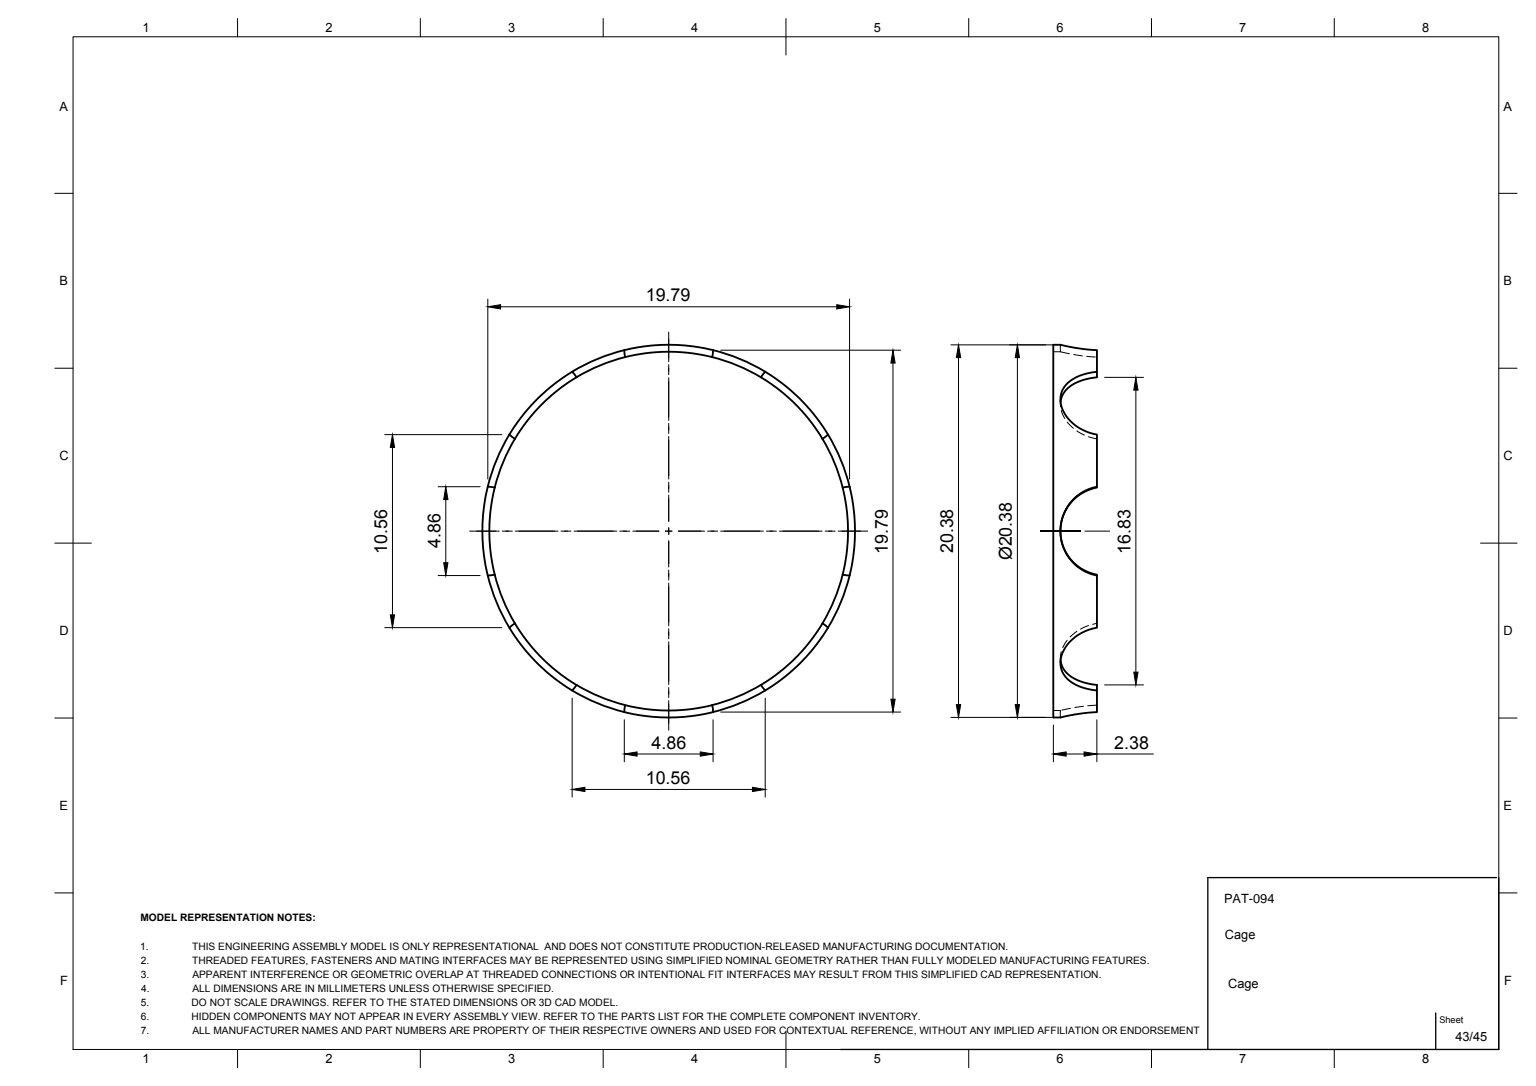
ISO-10303-21;
HEADER;
/* Generated by software containing ST-Developer
 * from STEP Tools, Inc. (www.steptools.com) 
 */

FILE_DESCRIPTION(
/* description */ ('Shaft runout checking stand'),
/* implementation_level */ '2;1');

FILE_NAME(
/* name */ 'Cage.step',
/* time_stamp */ '2026-11-02T21:12:33-08:00',
/* author */ (''),
/* organization */ (''),
/* preprocessor_version */ 'ST-DEVELOPER v20.2',
/* originating_system */ 'Autodesk Translation Framework v15.17.0.0',
/* authorisation */ '');

FILE_SCHEMA (('AUTOMOTIVE_DESIGN { 1 0 10303 214 3 1 1 }'));
ENDSEC;

DATA;
#10=MECHANICAL_DESIGN_GEOMETRIC_PRESENTATION_REPRESENTATION('',(#508),#11748);
#19=SPHERICAL_SURFACE('',#7380,0.247676);
#20=SPHERICAL_SURFACE('',#7396,0.247676);
#21=SPHERICAL_SURFACE('',#7401,0.247676);
#22=SPHERICAL_SURFACE('',#7406,0.247676);
#23=SPHERICAL_SURFACE('',#7411,0.247676);
#24=SPHERICAL_SURFACE('',#7416,0.247676);
#25=SPHERICAL_SURFACE('',#7421,0.247676);
#26=SPHERICAL_SURFACE('',#7429,0.247676);
#335=B_SPLINE_CURVE_WITH_KNOTS('',3,(#11118,#11119,#11120,#11121,#11122,
#11123,#11124,#11125,#11126,#11127,#11128,#11129,#11130,#11131,#11132,#11133,
#11134,#11135,#11136,#11137,#11138,#11139),.UNSPECIFIED.,.F.,.F.,(4,2,2,
2,2,2,2,2,2,2,4),(0.0473477652366656,0.126350602536658,0.189525903804987,
0.252701205073317,0.313298422430275,0.373895639787233,0.434492857144191,
0.495090074501149,0.558265375769478,0.621440677037807,0.7004435143378),
 .UNSPECIFIED.);
#336=B_SPLINE_CURVE_WITH_KNOTS('',3,(#11143,#11144,#11145,#11146,#11147,
#11148,#11149,#11150,#11151,#11152,#11153,#11154,#11155,#11156,#11157,#11158,
#11159,#11160,#11161,#11162,#11163,#11164),.UNSPECIFIED.,.F.,.F.,(4,2,2,
2,2,2,2,2,2,2,4),(0.0464897534940957,0.0852567806515119,0.170513561303024,
0.246687263103517,0.308657850341199,0.370628437578881,0.432599024816563,
0.494569612054245,0.570743313854739,0.656000094506251,0.694767121663666),
 .UNSPECIFIED.);
#337=B_SPLINE_CURVE_WITH_KNOTS('',3,(#11170,#11171,#11172,#11173,#11174,
#11175,#11176,#11177,#11178,#11179,#11180,#11181,#11182,#11183,#11184,#11185,
#11186,#11187,#11188,#11189,#11190,#11191),.UNSPECIFIED.,.F.,.F.,(4,2,2,
2,2,2,2,2,2,2,4),(0.0464897534940957,0.0852567806515118,0.170513561303024,
0.246687263103517,0.308657850341199,0.370628437578881,0.432599024816563,
0.494569612054245,0.570743313854738,0.65600009450625,0.694767121663666),
 .UNSPECIFIED.);
#338=B_SPLINE_CURVE_WITH_KNOTS('',3,(#11195,#11196,#11197,#11198,#11199,
#11200,#11201,#11202,#11203,#11204,#11205,#11206,#11207,#11208,#11209,#11210,
#11211,#11212,#11213,#11214,#11215,#11216),.UNSPECIFIED.,.F.,.F.,(4,2,2,
2,2,2,2,2,2,2,4),(0.0464897534940957,0.0852567806515119,0.170513561303024,
0.246687263103517,0.308657850341199,0.370628437578881,0.432599024816563,
0.494569612054245,0.570743313854739,0.656000094506251,0.694767121663666),
 .UNSPECIFIED.);
#339=B_SPLINE_CURVE_WITH_KNOTS('',3,(#11220,#11221,#11222,#11223,#11224,
#11225,#11226,#11227,#11228,#11229,#11230,#11231),.UNSPECIFIED.,.F.,.F.,
(4,2,2,2,2,4),(0.0464897534940957,0.0852567806515119,0.170513561303024,
0.246687263103517,0.308657850341199,0.370628437578881),.UNSPECIFIED.);
#340=B_SPLINE_CURVE_WITH_KNOTS('',3,(#11236,#11237,#11238,#11239,#11240,
#11241,#11242,#11243,#11244,#11245,#11246,#11247),.UNSPECIFIED.,.F.,.F.,
(4,2,2,2,2,4),(0.370628437578881,0.432599024816563,0.494569612054245,0.570743313854738,
0.65600009450625,0.694767121663666),.UNSPECIFIED.);
#341=B_SPLINE_CURVE_WITH_KNOTS('',3,(#11251,#11252,#11253,#11254,#11255,
#11256,#11257,#11258,#11259,#11260,#11261,#11262,#11263,#11264,#11265,#11266,
#11267,#11268,#11269,#11270,#11271,#11272),.UNSPECIFIED.,.F.,.F.,(4,2,2,
2,2,2,2,2,2,2,4),(0.0464897534940957,0.0852567806515121,0.170513561303024,
0.246687263103518,0.308657850341199,0.370628437578881,0.432599024816563,
0.494569612054245,0.570743313854738,0.65600009450625,0.694767121663666),
 .UNSPECIFIED.);
#342=B_SPLINE_CURVE_WITH_KNOTS('',3,(#11276,#11277,#11278,#11279,#11280,
#11281,#11282,#11283,#11284,#11285,#11286,#11287,#11288,#11289,#11290,#11291,
#11292,#11293,#11294,#11295,#11296,#11297),.UNSPECIFIED.,.F.,.F.,(4,2,2,
2,2,2,2,2,2,2,4),(0.0464897534940957,0.0852567806515119,0.170513561303024,
0.246687263103517,0.308657850341199,0.370628437578881,0.432599024816563,
0.494569612054245,0.570743313854738,0.65600009450625,0.694767121663667),
 .UNSPECIFIED.);
#343=B_SPLINE_CURVE_WITH_KNOTS('',3,(#11301,#11302,#11303,#11304,#11305,
#11306,#11307,#11308,#11309,#11310,#11311,#11312,#11313,#11314,#11315,#11316,
#11317,#11318,#11319,#11320,#11321,#11322),.UNSPECIFIED.,.F.,.F.,(4,2,2,
2,2,2,2,2,2,2,4),(0.0464897534940957,0.0852567806515119,0.170513561303024,
0.246687263103517,0.308657850341199,0.370628437578881,0.432599024816563,
0.494569612054245,0.570743313854738,0.65600009450625,0.694767121663666),
 .UNSPECIFIED.);
#344=B_SPLINE_CURVE_WITH_KNOTS('',3,(#11326,#11327,#11328,#11329,#11330,
#11331,#11332,#11333,#11334,#11335,#11336,#11337,#11338,#11339,#11340,#11341,
#11342,#11343,#11344,#11345,#11346,#11347),.UNSPECIFIED.,.F.,.F.,(4,2,2,
2,2,2,2,2,2,2,4),(0.0464897534940957,0.0852567806515119,0.170513561303024,
0.246687263103517,0.308657850341199,0.370628437578881,0.432599024816563,
0.494569612054245,0.570743313854739,0.656000094506251,0.694767121663667),
 .UNSPECIFIED.);
#345=B_SPLINE_CURVE_WITH_KNOTS('',3,(#11355,#11356,#11357,#11358,#11359,
#11360,#11361,#11362,#11363,#11364,#11365,#11366,#11367,#11368,#11369,#11370,
#11371,#11372,#11373,#11374,#11375,#11376),.UNSPECIFIED.,.F.,.F.,(4,2,2,
2,2,2,2,2,2,2,4),(0.0473477652366656,0.126350602536658,0.189525903804987,
0.252701205073316,0.313298422430274,0.373895639787232,0.434492857144191,
0.495090074501149,0.558265375769478,0.621440677037807,0.7004435143378),
 .UNSPECIFIED.);
#346=B_SPLINE_CURVE_WITH_KNOTS('',3,(#11384,#11385,#11386,#11387,#11388,
#11389,#11390,#11391,#11392,#11393,#11394,#11395,#11396,#11397,#11398,#11399,
#11400,#11401,#11402,#11403,#11404,#11405),.UNSPECIFIED.,.F.,.F.,(4,2,2,
2,2,2,2,2,2,2,4),(0.0473477652366656,0.126350602536658,0.189525903804987,
0.252701205073317,0.313298422430275,0.373895639787233,0.434492857144191,
0.495090074501149,0.558265375769478,0.621440677037807,0.7004435143378),
 .UNSPECIFIED.);
#347=B_SPLINE_CURVE_WITH_KNOTS('',3,(#11414,#11415,#11416,#11417,#11418,
#11419,#11420,#11421,#11422,#11423,#11424,#11425),.UNSPECIFIED.,.F.,.F.,
(4,2,2,2,2,4),(0.0473477652366656,0.126350602536658,0.189525903804987,0.252701205073316,
0.313298422430275,0.373895639787233),.UNSPECIFIED.);
#348=B_SPLINE_CURVE_WITH_KNOTS('',3,(#11427,#11428,#11429,#11430,#11431,
#11432,#11433,#11434,#11435,#11436,#11437,#11438),.UNSPECIFIED.,.F.,.F.,
(4,2,2,2,2,4),(0.373895639787233,0.434492857144191,0.495090074501149,0.558265375769478,
0.621440677037807,0.7004435143378),.UNSPECIFIED.);
#349=B_SPLINE_CURVE_WITH_KNOTS('',3,(#11445,#11446,#11447,#11448,#11449,
#11450,#11451,#11452,#11453,#11454,#11455,#11456,#11457,#11458,#11459,#11460,
#11461,#11462,#11463,#11464,#11465,#11466),.UNSPECIFIED.,.F.,.F.,(4,2,2,
2,2,2,2,2,2,2,4),(0.0473477652366656,0.126350602536658,0.189525903804987,
0.252701205073316,0.313298422430275,0.373895639787233,0.434492857144191,
0.495090074501149,0.558265375769478,0.621440677037807,0.7004435143378),
 .UNSPECIFIED.);
#350=B_SPLINE_CURVE_WITH_KNOTS('',3,(#11474,#11475,#11476,#11477,#11478,
#11479,#11480,#11481,#11482,#11483,#11484,#11485,#11486,#11487,#11488,#11489,
#11490,#11491,#11492,#11493,#11494,#11495),.UNSPECIFIED.,.F.,.F.,(4,2,2,
2,2,2,2,2,2,2,4),(0.0473477652366656,0.126350602536658,0.189525903804987,
0.252701205073317,0.313298422430275,0.373895639787233,0.434492857144191,
0.495090074501149,0.558265375769478,0.621440677037807,0.7004435143378),
 .UNSPECIFIED.);
#351=B_SPLINE_CURVE_WITH_KNOTS('',3,(#11503,#11504,#11505,#11506,#11507,
#11508,#11509,#11510,#11511,#11512,#11513,#11514,#11515,#11516,#11517,#11518,
#11519,#11520,#11521,#11522,#11523,#11524),.UNSPECIFIED.,.F.,.F.,(4,2,2,
2,2,2,2,2,2,2,4),(0.0473477652366656,0.126350602536658,0.189525903804987,
0.252701205073316,0.313298422430275,0.373895639787233,0.434492857144191,
0.495090074501149,0.558265375769478,0.621440677037807,0.7004435143378),
 .UNSPECIFIED.);
#352=B_SPLINE_CURVE_WITH_KNOTS('',3,(#11533,#11534,#11535,#11536,#11537,
#11538,#11539,#11540,#11541,#11542,#11543,#11544,#11545,#11546,#11547,#11548,
#11549,#11550,#11551,#11552,#11553,#11554),.UNSPECIFIED.,.F.,.F.,(4,2,2,
2,2,2,2,2,2,2,4),(0.0473477652366656,0.126350602536658,0.189525903804987,
0.252701205073317,0.313298422430275,0.373895639787233,0.434492857144191,
0.495090074501149,0.558265375769478,0.621440677037807,0.7004435143378),
 .UNSPECIFIED.);
#415=SHAPE_REPRESENTATION_RELATIONSHIP('SRR','None',#11967,#458);
#458=ADVANCED_BREP_SHAPE_REPRESENTATION('',(#556),#11743);
#508=STYLED_ITEM('',(#12169),#556);
#556=MANIFOLD_SOLID_BREP('Continuous crown cage',#6254);
#662=FACE_BOUND('',#1853,.T.);
#884=CIRCLE('',#7381,0.243053047864041);
#885=CIRCLE('',#7382,0.243053047864041);
#886=CIRCLE('',#7384,1.019052);
#887=CIRCLE('',#7385,1.019052);
#888=CIRCLE('',#7386,1.019052);
#889=CIRCLE('',#7387,1.019052);
#890=CIRCLE('',#7388,1.019052);
#891=CIRCLE('',#7389,1.019052);
#892=CIRCLE('',#7390,1.019052);
#893=CIRCLE('',#7391,1.019052);
#894=CIRCLE('',#7392,1.019052);
#895=CIRCLE('',#7394,0.980948);
#896=CIRCLE('',#7395,0.243053047864041);
#897=CIRCLE('',#7397,0.243053047864041);
#898=CIRCLE('',#7399,0.980948);
#899=CIRCLE('',#7400,0.243053047864041);
#900=CIRCLE('',#7402,0.243053047864041);
#901=CIRCLE('',#7404,0.980948);
#902=CIRCLE('',#7405,0.243053047864041);
#903=CIRCLE('',#7407,0.243053047864041);
#904=CIRCLE('',#7409,0.980948);
#905=CIRCLE('',#7410,0.243053047864041);
#906=CIRCLE('',#7412,0.243053047864041);
#907=CIRCLE('',#7414,0.980948);
#908=CIRCLE('',#7415,0.243053047864041);
#909=CIRCLE('',#7417,0.243053047864041);
#910=CIRCLE('',#7419,0.980948);
#911=CIRCLE('',#7420,0.243053047864041);
#912=CIRCLE('',#7422,0.243053047864041);
#913=CIRCLE('',#7424,0.980948);
#914=CIRCLE('',#7425,0.980948);
#915=CIRCLE('',#7426,0.980948);
#916=CIRCLE('',#7428,0.243053047864041);
#917=CIRCLE('',#7430,0.243053047864041);
#1026=CYLINDRICAL_SURFACE('',#7383,1.019052);
#1027=CYLINDRICAL_SURFACE('',#7423,0.980948);
#1367=FACE_OUTER_BOUND('',#1835,.T.);
#1368=FACE_OUTER_BOUND('',#1836,.T.);
#1369=FACE_OUTER_BOUND('',#1837,.T.);
#1370=FACE_OUTER_BOUND('',#1838,.T.);
#1371=FACE_OUTER_BOUND('',#1839,.T.);
#1372=FACE_OUTER_BOUND('',#1840,.T.);
#1373=FACE_OUTER_BOUND('',#1841,.T.);
#1374=FACE_OUTER_BOUND('',#1842,.T.);
#1375=FACE_OUTER_BOUND('',#1843,.T.);
#1376=FACE_OUTER_BOUND('',#1844,.T.);
#1377=FACE_OUTER_BOUND('',#1845,.T.);
#1378=FACE_OUTER_BOUND('',#1846,.T.);
#1379=FACE_OUTER_BOUND('',#1847,.T.);
#1380=FACE_OUTER_BOUND('',#1848,.T.);
#1381=FACE_OUTER_BOUND('',#1849,.T.);
#1382=FACE_OUTER_BOUND('',#1850,.T.);
#1383=FACE_OUTER_BOUND('',#1851,.T.);
#1384=FACE_OUTER_BOUND('',#1852,.T.);
#1385=FACE_OUTER_BOUND('',#1854,.T.);
#1835=EDGE_LOOP('',(#5436,#5437,#5438,#5439));
#1836=EDGE_LOOP('',(#5440,#5441,#5442,#5443,#5444,#5445,#5446,#5447,#5448,
#5449,#5450,#5451,#5452,#5453,#5454,#5455,#5456,#5457,#5458,#5459));
#1837=EDGE_LOOP('',(#5460,#5461,#5462,#5463));
#1838=EDGE_LOOP('',(#5464,#5465,#5466,#5467));
#1839=EDGE_LOOP('',(#5468,#5469,#5470,#5471));
#1840=EDGE_LOOP('',(#5472,#5473,#5474,#5475));
#1841=EDGE_LOOP('',(#5476,#5477,#5478,#5479));
#1842=EDGE_LOOP('',(#5480,#5481,#5482,#5483,#5484,#5485));
#1843=EDGE_LOOP('',(#5486,#5487,#5488,#5489));
#1844=EDGE_LOOP('',(#5490,#5491,#5492,#5493));
#1845=EDGE_LOOP('',(#5494,#5495,#5496,#5497));
#1846=EDGE_LOOP('',(#5498,#5499,#5500,#5501));
#1847=EDGE_LOOP('',(#5502,#5503,#5504,#5505));
#1848=EDGE_LOOP('',(#5506,#5507,#5508,#5509));
#1849=EDGE_LOOP('',(#5510,#5511,#5512,#5513,#5514,#5515,#5516,#5517,#5518,
#5519,#5520,#5521,#5522,#5523,#5524,#5525,#5526,#5527,#5528,#5529));
#1850=EDGE_LOOP('',(#5530,#5531,#5532,#5533));
#1851=EDGE_LOOP('',(#5534,#5535,#5536,#5537));
#1852=EDGE_LOOP('',(#5538));
#1853=EDGE_LOOP('',(#5539));
#1854=EDGE_LOOP('',(#5540,#5541,#5542,#5543));
#2340=LINE('',#11233,#2807);
#2341=LINE('',#11529,#2808);
#2807=VECTOR('',#9253,1.019052);
#2808=VECTOR('',#9330,0.980948);
#3274=VERTEX_POINT('',#11116);
#3275=VERTEX_POINT('',#11117);
#3276=VERTEX_POINT('',#11140);
#3277=VERTEX_POINT('',#11142);
#3278=VERTEX_POINT('',#11167);
#3279=VERTEX_POINT('',#11169);
#3280=VERTEX_POINT('',#11192);
#3281=VERTEX_POINT('',#11194);
#3282=VERTEX_POINT('',#11217);
#3283=VERTEX_POINT('',#11219);
#3284=VERTEX_POINT('',#11232);
#3285=VERTEX_POINT('',#11235);
#3286=VERTEX_POINT('',#11248);
#3287=VERTEX_POINT('',#11250);
#3288=VERTEX_POINT('',#11273);
#3289=VERTEX_POINT('',#11275);
#3290=VERTEX_POINT('',#11298);
#3291=VERTEX_POINT('',#11300);
#3292=VERTEX_POINT('',#11323);
#3293=VERTEX_POINT('',#11325);
#3294=VERTEX_POINT('',#11350);
#3295=VERTEX_POINT('',#11354);
#3296=VERTEX_POINT('',#11379);
#3297=VERTEX_POINT('',#11383);
#3298=VERTEX_POINT('',#11408);
#3299=VERTEX_POINT('',#11412);
#3300=VERTEX_POINT('',#11413);
#3301=VERTEX_POINT('',#11440);
#3302=VERTEX_POINT('',#11444);
#3303=VERTEX_POINT('',#11469);
#3304=VERTEX_POINT('',#11473);
#3305=VERTEX_POINT('',#11498);
#3306=VERTEX_POINT('',#11502);
#3307=VERTEX_POINT('',#11527);
#3308=VERTEX_POINT('',#11530);
#3309=VERTEX_POINT('',#11532);
#4004=EDGE_CURVE('',#3274,#3275,#335,.T.);
#4005=EDGE_CURVE('',#3276,#3274,#884,.T.);
#4006=EDGE_CURVE('',#3277,#3276,#336,.T.);
#4007=EDGE_CURVE('',#3275,#3277,#885,.T.);
#4008=EDGE_CURVE('',#3278,#3276,#886,.T.);
#4009=EDGE_CURVE('',#3278,#3279,#337,.T.);
#4010=EDGE_CURVE('',#3280,#3279,#887,.T.);
#4011=EDGE_CURVE('',#3280,#3281,#338,.T.);
#4012=EDGE_CURVE('',#3282,#3281,#888,.T.);
#4013=EDGE_CURVE('',#3282,#3283,#339,.T.);
#4014=EDGE_CURVE('',#3283,#3284,#2340,.T.);
#4015=EDGE_CURVE('',#3284,#3284,#889,.T.);
#4016=EDGE_CURVE('',#3283,#3285,#340,.T.);
#4017=EDGE_CURVE('',#3286,#3285,#890,.T.);
#4018=EDGE_CURVE('',#3286,#3287,#341,.T.);
#4019=EDGE_CURVE('',#3288,#3287,#891,.T.);
#4020=EDGE_CURVE('',#3288,#3289,#342,.T.);
#4021=EDGE_CURVE('',#3290,#3289,#892,.T.);
#4022=EDGE_CURVE('',#3290,#3291,#343,.T.);
#4023=EDGE_CURVE('',#3292,#3291,#893,.T.);
#4024=EDGE_CURVE('',#3292,#3293,#344,.T.);
#4025=EDGE_CURVE('',#3277,#3293,#894,.T.);
#4026=EDGE_CURVE('',#3274,#3294,#895,.T.);
#4027=EDGE_CURVE('',#3294,#3278,#896,.T.);
#4028=EDGE_CURVE('',#3295,#3294,#345,.T.);
#4029=EDGE_CURVE('',#3279,#3295,#897,.T.);
#4030=EDGE_CURVE('',#3295,#3296,#898,.T.);
#4031=EDGE_CURVE('',#3296,#3280,#899,.T.);
#4032=EDGE_CURVE('',#3297,#3296,#346,.T.);
#4033=EDGE_CURVE('',#3281,#3297,#900,.T.);
#4034=EDGE_CURVE('',#3297,#3298,#901,.T.);
#4035=EDGE_CURVE('',#3298,#3282,#902,.T.);
#4036=EDGE_CURVE('',#3299,#3300,#347,.T.);
#4037=EDGE_CURVE('',#3285,#3299,#903,.T.);
#4038=EDGE_CURVE('',#3300,#3298,#348,.T.);
#4039=EDGE_CURVE('',#3299,#3301,#904,.T.);
#4040=EDGE_CURVE('',#3301,#3286,#905,.T.);
#4041=EDGE_CURVE('',#3302,#3301,#349,.T.);
#4042=EDGE_CURVE('',#3287,#3302,#906,.T.);
#4043=EDGE_CURVE('',#3302,#3303,#907,.T.);
#4044=EDGE_CURVE('',#3303,#3288,#908,.T.);
#4045=EDGE_CURVE('',#3304,#3303,#350,.T.);
#4046=EDGE_CURVE('',#3289,#3304,#909,.T.);
#4047=EDGE_CURVE('',#3304,#3305,#910,.T.);
#4048=EDGE_CURVE('',#3305,#3290,#911,.T.);
#4049=EDGE_CURVE('',#3306,#3305,#351,.T.);
#4050=EDGE_CURVE('',#3291,#3306,#912,.T.);
#4051=EDGE_CURVE('',#3307,#3307,#913,.T.);
#4052=EDGE_CURVE('',#3307,#3300,#2341,.T.);
#4053=EDGE_CURVE('',#3308,#3275,#914,.T.);
#4054=EDGE_CURVE('',#3308,#3309,#352,.T.);
#4055=EDGE_CURVE('',#3306,#3309,#915,.T.);
#4056=EDGE_CURVE('',#3293,#3308,#916,.T.);
#4057=EDGE_CURVE('',#3309,#3292,#917,.T.);
#5436=ORIENTED_EDGE('',*,*,#4004,.F.);
#5437=ORIENTED_EDGE('',*,*,#4005,.F.);
#5438=ORIENTED_EDGE('',*,*,#4006,.F.);
#5439=ORIENTED_EDGE('',*,*,#4007,.F.);
#5440=ORIENTED_EDGE('',*,*,#4006,.T.);
#5441=ORIENTED_EDGE('',*,*,#4008,.F.);
#5442=ORIENTED_EDGE('',*,*,#4009,.T.);
#5443=ORIENTED_EDGE('',*,*,#4010,.F.);
#5444=ORIENTED_EDGE('',*,*,#4011,.T.);
#5445=ORIENTED_EDGE('',*,*,#4012,.F.);
#5446=ORIENTED_EDGE('',*,*,#4013,.T.);
#5447=ORIENTED_EDGE('',*,*,#4014,.T.);
#5448=ORIENTED_EDGE('',*,*,#4015,.F.);
#5449=ORIENTED_EDGE('',*,*,#4014,.F.);
#5450=ORIENTED_EDGE('',*,*,#4016,.T.);
#5451=ORIENTED_EDGE('',*,*,#4017,.F.);
#5452=ORIENTED_EDGE('',*,*,#4018,.T.);
#5453=ORIENTED_EDGE('',*,*,#4019,.F.);
#5454=ORIENTED_EDGE('',*,*,#4020,.T.);
#5455=ORIENTED_EDGE('',*,*,#4021,.F.);
#5456=ORIENTED_EDGE('',*,*,#4022,.T.);
#5457=ORIENTED_EDGE('',*,*,#4023,.F.);
#5458=ORIENTED_EDGE('',*,*,#4024,.T.);
#5459=ORIENTED_EDGE('',*,*,#4025,.F.);
#5460=ORIENTED_EDGE('',*,*,#4005,.T.);
#5461=ORIENTED_EDGE('',*,*,#4026,.T.);
#5462=ORIENTED_EDGE('',*,*,#4027,.T.);
#5463=ORIENTED_EDGE('',*,*,#4008,.T.);
#5464=ORIENTED_EDGE('',*,*,#4028,.F.);
#5465=ORIENTED_EDGE('',*,*,#4029,.F.);
#5466=ORIENTED_EDGE('',*,*,#4009,.F.);
#5467=ORIENTED_EDGE('',*,*,#4027,.F.);
#5468=ORIENTED_EDGE('',*,*,#4029,.T.);
#5469=ORIENTED_EDGE('',*,*,#4030,.T.);
#5470=ORIENTED_EDGE('',*,*,#4031,.T.);
#5471=ORIENTED_EDGE('',*,*,#4010,.T.);
#5472=ORIENTED_EDGE('',*,*,#4032,.F.);
#5473=ORIENTED_EDGE('',*,*,#4033,.F.);
#5474=ORIENTED_EDGE('',*,*,#4011,.F.);
#5475=ORIENTED_EDGE('',*,*,#4031,.F.);
#5476=ORIENTED_EDGE('',*,*,#4033,.T.);
#5477=ORIENTED_EDGE('',*,*,#4034,.T.);
#5478=ORIENTED_EDGE('',*,*,#4035,.T.);
#5479=ORIENTED_EDGE('',*,*,#4012,.T.);
#5480=ORIENTED_EDGE('',*,*,#4036,.F.);
#5481=ORIENTED_EDGE('',*,*,#4037,.F.);
#5482=ORIENTED_EDGE('',*,*,#4016,.F.);
#5483=ORIENTED_EDGE('',*,*,#4013,.F.);
#5484=ORIENTED_EDGE('',*,*,#4035,.F.);
#5485=ORIENTED_EDGE('',*,*,#4038,.F.);
#5486=ORIENTED_EDGE('',*,*,#4037,.T.);
#5487=ORIENTED_EDGE('',*,*,#4039,.T.);
#5488=ORIENTED_EDGE('',*,*,#4040,.T.);
#5489=ORIENTED_EDGE('',*,*,#4017,.T.);
#5490=ORIENTED_EDGE('',*,*,#4041,.F.);
#5491=ORIENTED_EDGE('',*,*,#4042,.F.);
#5492=ORIENTED_EDGE('',*,*,#4018,.F.);
#5493=ORIENTED_EDGE('',*,*,#4040,.F.);
#5494=ORIENTED_EDGE('',*,*,#4042,.T.);
#5495=ORIENTED_EDGE('',*,*,#4043,.T.);
#5496=ORIENTED_EDGE('',*,*,#4044,.T.);
#5497=ORIENTED_EDGE('',*,*,#4019,.T.);
#5498=ORIENTED_EDGE('',*,*,#4045,.F.);
#5499=ORIENTED_EDGE('',*,*,#4046,.F.);
#5500=ORIENTED_EDGE('',*,*,#4020,.F.);
#5501=ORIENTED_EDGE('',*,*,#4044,.F.);
#5502=ORIENTED_EDGE('',*,*,#4046,.T.);
#5503=ORIENTED_EDGE('',*,*,#4047,.T.);
#5504=ORIENTED_EDGE('',*,*,#4048,.T.);
#5505=ORIENTED_EDGE('',*,*,#4021,.T.);
#5506=ORIENTED_EDGE('',*,*,#4022,.F.);
#5507=ORIENTED_EDGE('',*,*,#4048,.F.);
#5508=ORIENTED_EDGE('',*,*,#4049,.F.);
#5509=ORIENTED_EDGE('',*,*,#4050,.F.);
#5510=ORIENTED_EDGE('',*,*,#4051,.F.);
#5511=ORIENTED_EDGE('',*,*,#4052,.T.);
#5512=ORIENTED_EDGE('',*,*,#4038,.T.);
#5513=ORIENTED_EDGE('',*,*,#4034,.F.);
#5514=ORIENTED_EDGE('',*,*,#4032,.T.);
#5515=ORIENTED_EDGE('',*,*,#4030,.F.);
#5516=ORIENTED_EDGE('',*,*,#4028,.T.);
#5517=ORIENTED_EDGE('',*,*,#4026,.F.);
#5518=ORIENTED_EDGE('',*,*,#4004,.T.);
#5519=ORIENTED_EDGE('',*,*,#4053,.F.);
#5520=ORIENTED_EDGE('',*,*,#4054,.T.);
#5521=ORIENTED_EDGE('',*,*,#4055,.F.);
#5522=ORIENTED_EDGE('',*,*,#4049,.T.);
#5523=ORIENTED_EDGE('',*,*,#4047,.F.);
#5524=ORIENTED_EDGE('',*,*,#4045,.T.);
#5525=ORIENTED_EDGE('',*,*,#4043,.F.);
#5526=ORIENTED_EDGE('',*,*,#4041,.T.);
#5527=ORIENTED_EDGE('',*,*,#4039,.F.);
#5528=ORIENTED_EDGE('',*,*,#4036,.T.);
#5529=ORIENTED_EDGE('',*,*,#4052,.F.);
#5530=ORIENTED_EDGE('',*,*,#4007,.T.);
#5531=ORIENTED_EDGE('',*,*,#4025,.T.);
#5532=ORIENTED_EDGE('',*,*,#4056,.T.);
#5533=ORIENTED_EDGE('',*,*,#4053,.T.);
#5534=ORIENTED_EDGE('',*,*,#4024,.F.);
#5535=ORIENTED_EDGE('',*,*,#4057,.F.);
#5536=ORIENTED_EDGE('',*,*,#4054,.F.);
#5537=ORIENTED_EDGE('',*,*,#4056,.F.);
#5538=ORIENTED_EDGE('',*,*,#4015,.T.);
#5539=ORIENTED_EDGE('',*,*,#4051,.T.);
#5540=ORIENTED_EDGE('',*,*,#4050,.T.);
#5541=ORIENTED_EDGE('',*,*,#4055,.T.);
#5542=ORIENTED_EDGE('',*,*,#4057,.T.);
#5543=ORIENTED_EDGE('',*,*,#4023,.T.);
#5819=PLANE('',#7393);
#5820=PLANE('',#7398);
#5821=PLANE('',#7403);
#5822=PLANE('',#7408);
#5823=PLANE('',#7413);
#5824=PLANE('',#7418);
#5825=PLANE('',#7427);
#5826=PLANE('',#7431);
#5827=PLANE('',#7432);
#6167=ADVANCED_FACE('',(#1367),#19,.F.);
#6168=ADVANCED_FACE('',(#1368),#1026,.T.);
#6169=ADVANCED_FACE('',(#1369),#5819,.T.);
#6170=ADVANCED_FACE('',(#1370),#20,.F.);
#6171=ADVANCED_FACE('',(#1371),#5820,.T.);
#6172=ADVANCED_FACE('',(#1372),#21,.F.);
#6173=ADVANCED_FACE('',(#1373),#5821,.T.);
#6174=ADVANCED_FACE('',(#1374),#22,.F.);
#6175=ADVANCED_FACE('',(#1375),#5822,.T.);
#6176=ADVANCED_FACE('',(#1376),#23,.F.);
#6177=ADVANCED_FACE('',(#1377),#5823,.T.);
#6178=ADVANCED_FACE('',(#1378),#24,.F.);
#6179=ADVANCED_FACE('',(#1379),#5824,.T.);
#6180=ADVANCED_FACE('',(#1380),#25,.F.);
#6181=ADVANCED_FACE('',(#1381),#1027,.F.);
#6182=ADVANCED_FACE('',(#1382),#5825,.T.);
#6183=ADVANCED_FACE('',(#1383),#26,.F.);
#6184=ADVANCED_FACE('',(#1384,#662),#5826,.T.);
#6185=ADVANCED_FACE('',(#1385),#5827,.T.);
#6254=CLOSED_SHELL('',(#6167,#6168,#6169,#6170,#6171,#6172,#6173,#6174,
#6175,#6176,#6177,#6178,#6179,#6180,#6181,#6182,#6183,#6184,#6185));
#7379=AXIS2_PLACEMENT_3D('',#11114,#9237,#9238);
#7380=AXIS2_PLACEMENT_3D('',#11115,#9239,#9240);
#7381=AXIS2_PLACEMENT_3D('',#11141,#9241,#9242);
#7382=AXIS2_PLACEMENT_3D('',#11165,#9243,#9244);
#7383=AXIS2_PLACEMENT_3D('',#11166,#9245,#9246);
#7384=AXIS2_PLACEMENT_3D('',#11168,#9247,#9248);
#7385=AXIS2_PLACEMENT_3D('',#11193,#9249,#9250);
#7386=AXIS2_PLACEMENT_3D('',#11218,#9251,#9252);
#7387=AXIS2_PLACEMENT_3D('',#11234,#9254,#9255);
#7388=AXIS2_PLACEMENT_3D('',#11249,#9256,#9257);
#7389=AXIS2_PLACEMENT_3D('',#11274,#9258,#9259);
#7390=AXIS2_PLACEMENT_3D('',#11299,#9260,#9261);
#7391=AXIS2_PLACEMENT_3D('',#11324,#9262,#9263);
#7392=AXIS2_PLACEMENT_3D('',#11348,#9264,#9265);
#7393=AXIS2_PLACEMENT_3D('',#11349,#9266,#9267);
#7394=AXIS2_PLACEMENT_3D('',#11351,#9268,#9269);
#7395=AXIS2_PLACEMENT_3D('',#11352,#9270,#9271);
#7396=AXIS2_PLACEMENT_3D('',#11353,#9272,#9273);
#7397=AXIS2_PLACEMENT_3D('',#11377,#9274,#9275);
#7398=AXIS2_PLACEMENT_3D('',#11378,#9276,#9277);
#7399=AXIS2_PLACEMENT_3D('',#11380,#9278,#9279);
#7400=AXIS2_PLACEMENT_3D('',#11381,#9280,#9281);
#7401=AXIS2_PLACEMENT_3D('',#11382,#9282,#9283);
#7402=AXIS2_PLACEMENT_3D('',#11406,#9284,#9285);
#7403=AXIS2_PLACEMENT_3D('',#11407,#9286,#9287);
#7404=AXIS2_PLACEMENT_3D('',#11409,#9288,#9289);
#7405=AXIS2_PLACEMENT_3D('',#11410,#9290,#9291);
#7406=AXIS2_PLACEMENT_3D('',#11411,#9292,#9293);
#7407=AXIS2_PLACEMENT_3D('',#11426,#9294,#9295);
#7408=AXIS2_PLACEMENT_3D('',#11439,#9296,#9297);
#7409=AXIS2_PLACEMENT_3D('',#11441,#9298,#9299);
#7410=AXIS2_PLACEMENT_3D('',#11442,#9300,#9301);
#7411=AXIS2_PLACEMENT_3D('',#11443,#9302,#9303);
#7412=AXIS2_PLACEMENT_3D('',#11467,#9304,#9305);
#7413=AXIS2_PLACEMENT_3D('',#11468,#9306,#9307);
#7414=AXIS2_PLACEMENT_3D('',#11470,#9308,#9309);
#7415=AXIS2_PLACEMENT_3D('',#11471,#9310,#9311);
#7416=AXIS2_PLACEMENT_3D('',#11472,#9312,#9313);
#7417=AXIS2_PLACEMENT_3D('',#11496,#9314,#9315);
#7418=AXIS2_PLACEMENT_3D('',#11497,#9316,#9317);
#7419=AXIS2_PLACEMENT_3D('',#11499,#9318,#9319);
#7420=AXIS2_PLACEMENT_3D('',#11500,#9320,#9321);
#7421=AXIS2_PLACEMENT_3D('',#11501,#9322,#9323);
#7422=AXIS2_PLACEMENT_3D('',#11525,#9324,#9325);
#7423=AXIS2_PLACEMENT_3D('',#11526,#9326,#9327);
#7424=AXIS2_PLACEMENT_3D('',#11528,#9328,#9329);
#7425=AXIS2_PLACEMENT_3D('',#11531,#9331,#9332);
#7426=AXIS2_PLACEMENT_3D('',#11555,#9333,#9334);
#7427=AXIS2_PLACEMENT_3D('',#11556,#9335,#9336);
#7428=AXIS2_PLACEMENT_3D('',#11557,#9337,#9338);
#7429=AXIS2_PLACEMENT_3D('',#11558,#9339,#9340);
#7430=AXIS2_PLACEMENT_3D('',#11559,#9341,#9342);
#7431=AXIS2_PLACEMENT_3D('',#11560,#9343,#9344);
#7432=AXIS2_PLACEMENT_3D('',#11561,#9345,#9346);
#9237=DIRECTION('axis',(0.,0.,1.));
#9238=DIRECTION('refdir',(1.,0.,0.));
#9239=DIRECTION('center_axis',(0.,0.,1.));
#9240=DIRECTION('ref_axis',(1.,0.,0.));
#9241=DIRECTION('center_axis',(0.,-1.,0.));
#9242=DIRECTION('ref_axis',(0.,0.,-1.));
#9243=DIRECTION('center_axis',(0.,-1.,0.));
#9244=DIRECTION('ref_axis',(0.,0.,-1.));
#9245=DIRECTION('center_axis',(0.,1.,0.));
#9246=DIRECTION('ref_axis',(1.,0.,0.));
#9247=DIRECTION('center_axis',(0.,1.,0.));
#9248=DIRECTION('ref_axis',(1.,0.,0.));
#9249=DIRECTION('center_axis',(0.,1.,0.));
#9250=DIRECTION('ref_axis',(1.,0.,0.));
#9251=DIRECTION('center_axis',(0.,1.,0.));
#9252=DIRECTION('ref_axis',(1.,0.,0.));
#9253=DIRECTION('',(0.,-1.,0.));
#9254=DIRECTION('center_axis',(0.,-1.,0.));
#9255=DIRECTION('ref_axis',(1.,0.,0.));
#9256=DIRECTION('center_axis',(0.,1.,0.));
#9257=DIRECTION('ref_axis',(1.,0.,0.));
#9258=DIRECTION('center_axis',(0.,1.,0.));
#9259=DIRECTION('ref_axis',(1.,0.,0.));
#9260=DIRECTION('center_axis',(0.,1.,0.));
#9261=DIRECTION('ref_axis',(1.,0.,0.));
#9262=DIRECTION('center_axis',(0.,1.,0.));
#9263=DIRECTION('ref_axis',(1.,0.,0.));
#9264=DIRECTION('center_axis',(0.,1.,0.));
#9265=DIRECTION('ref_axis',(1.,0.,0.));
#9266=DIRECTION('center_axis',(0.,1.,0.));
#9267=DIRECTION('ref_axis',(1.,0.,0.));
#9268=DIRECTION('center_axis',(0.,-1.,0.));
#9269=DIRECTION('ref_axis',(1.,0.,0.));
#9270=DIRECTION('center_axis',(0.,-1.,0.));
#9271=DIRECTION('ref_axis',(0.,0.,-1.));
#9272=DIRECTION('center_axis',(6.12323399573677E-17,0.,1.));
#9273=DIRECTION('ref_axis',(1.,0.,0.));
#9274=DIRECTION('center_axis',(0.,-1.,0.));
#9275=DIRECTION('ref_axis',(0.,0.,-1.));
#9276=DIRECTION('center_axis',(0.,1.,0.));
#9277=DIRECTION('ref_axis',(1.,0.,0.));
#9278=DIRECTION('center_axis',(0.,-1.,0.));
#9279=DIRECTION('ref_axis',(1.,0.,0.));
#9280=DIRECTION('center_axis',(0.,-1.,0.));
#9281=DIRECTION('ref_axis',(0.,0.,-1.));
#9282=DIRECTION('center_axis',(0.,0.,1.));
#9283=DIRECTION('ref_axis',(1.,0.,0.));
#9284=DIRECTION('center_axis',(0.,-1.,0.));
#9285=DIRECTION('ref_axis',(0.,0.,-1.));
#9286=DIRECTION('center_axis',(0.,1.,0.));
#9287=DIRECTION('ref_axis',(1.,0.,0.));
#9288=DIRECTION('center_axis',(0.,-1.,0.));
#9289=DIRECTION('ref_axis',(1.,0.,0.));
#9290=DIRECTION('center_axis',(0.,-1.,0.));
#9291=DIRECTION('ref_axis',(0.,0.,-1.));
#9292=DIRECTION('center_axis',(0.,0.,1.));
#9293=DIRECTION('ref_axis',(1.,0.,0.));
#9294=DIRECTION('center_axis',(0.,-1.,0.));
#9295=DIRECTION('ref_axis',(0.,0.,-1.));
#9296=DIRECTION('center_axis',(0.,1.,0.));
#9297=DIRECTION('ref_axis',(1.,0.,0.));
#9298=DIRECTION('center_axis',(0.,-1.,0.));
#9299=DIRECTION('ref_axis',(1.,0.,0.));
#9300=DIRECTION('center_axis',(0.,-1.,0.));
#9301=DIRECTION('ref_axis',(0.,0.,-1.));
#9302=DIRECTION('center_axis',(0.,0.,1.));
#9303=DIRECTION('ref_axis',(1.,0.,0.));
#9304=DIRECTION('center_axis',(0.,-1.,0.));
#9305=DIRECTION('ref_axis',(0.,0.,-1.));
#9306=DIRECTION('center_axis',(0.,1.,0.));
#9307=DIRECTION('ref_axis',(1.,0.,0.));
#9308=DIRECTION('center_axis',(0.,-1.,0.));
#9309=DIRECTION('ref_axis',(1.,0.,0.));
#9310=DIRECTION('center_axis',(0.,-1.,0.));
#9311=DIRECTION('ref_axis',(0.,0.,-1.));
#9312=DIRECTION('center_axis',(6.12323399573676E-17,0.,1.));
#9313=DIRECTION('ref_axis',(1.,0.,0.));
#9314=DIRECTION('center_axis',(0.,-1.,0.));
#9315=DIRECTION('ref_axis',(0.,0.,-1.));
#9316=DIRECTION('center_axis',(0.,1.,0.));
#9317=DIRECTION('ref_axis',(1.,0.,0.));
#9318=DIRECTION('center_axis',(0.,-1.,0.));
#9319=DIRECTION('ref_axis',(1.,0.,0.));
#9320=DIRECTION('center_axis',(0.,-1.,0.));
#9321=DIRECTION('ref_axis',(0.,0.,-1.));
#9322=DIRECTION('center_axis',(0.,0.,1.));
#9323=DIRECTION('ref_axis',(1.,0.,0.));
#9324=DIRECTION('center_axis',(0.,-1.,0.));
#9325=DIRECTION('ref_axis',(0.,0.,-1.));
#9326=DIRECTION('center_axis',(0.,1.,0.));
#9327=DIRECTION('ref_axis',(1.,0.,0.));
#9328=DIRECTION('center_axis',(0.,1.,0.));
#9329=DIRECTION('ref_axis',(1.,0.,0.));
#9330=DIRECTION('',(0.,1.,0.));
#9331=DIRECTION('center_axis',(0.,-1.,0.));
#9332=DIRECTION('ref_axis',(1.,0.,0.));
#9333=DIRECTION('center_axis',(0.,-1.,0.));
#9334=DIRECTION('ref_axis',(1.,0.,0.));
#9335=DIRECTION('center_axis',(0.,1.,0.));
#9336=DIRECTION('ref_axis',(1.,0.,0.));
#9337=DIRECTION('center_axis',(0.,-1.,0.));
#9338=DIRECTION('ref_axis',(0.,0.,-1.));
#9339=DIRECTION('center_axis',(0.,0.,1.));
#9340=DIRECTION('ref_axis',(1.,0.,0.));
#9341=DIRECTION('center_axis',(0.,-1.,0.));
#9342=DIRECTION('ref_axis',(0.,0.,-1.));
#9343=DIRECTION('center_axis',(0.,-1.,0.));
#9344=DIRECTION('ref_axis',(-1.,0.,0.));
#9345=DIRECTION('center_axis',(0.,1.,0.));
#9346=DIRECTION('ref_axis',(1.,0.,0.));
#11114=CARTESIAN_POINT('',(0.,0.,0.));
#11115=CARTESIAN_POINT('Origin',(0.707106781186547,0.,0.707106781186548));
#11116=CARTESIAN_POINT('',(0.504455939115715,-0.04763,0.841298510752802));
#11117=CARTESIAN_POINT('',(0.841298510752802,-0.04763,0.504455939115715));
#11118=CARTESIAN_POINT('Ctrl Pts',(0.504455939115715,-0.04763,0.841298510752802));
#11119=CARTESIAN_POINT('Ctrl Pts',(0.508899795931835,-0.0740444353928835,
0.838633903678357));
#11120=CARTESIAN_POINT('Ctrl Pts',(0.517157748491652,-0.0999305678883309,
0.833661031856294));
#11121=CARTESIAN_POINT('Ctrl Pts',(0.537715343527944,-0.142345102874864,
0.820511285096538));
#11122=CARTESIAN_POINT('Ctrl Pts',(0.548874290046456,-0.159766064500479,
0.813159949759));
#11123=CARTESIAN_POINT('Ctrl Pts',(0.573915184558107,-0.190326085855194,
0.795684265985089));
#11124=CARTESIAN_POINT('Ctrl Pts',(0.587792702767295,-0.203463743702801,
0.78555112003688));
#11125=CARTESIAN_POINT('Ctrl Pts',(0.615966552324775,-0.224161999508995,
0.763642258217233));
#11126=CARTESIAN_POINT('Ctrl Pts',(0.631684198665438,-0.232861760990032,
0.750785745543687));
#11127=CARTESIAN_POINT('Ctrl Pts',(0.663382628119203,-0.244251601209411,
0.722929908501543));
#11128=CARTESIAN_POINT('Ctrl Pts',(0.679352081686668,-0.246942143572133,
0.707917883896095));
#11129=CARTESIAN_POINT('Ctrl Pts',(0.707917883896095,-0.246942143572133,
0.679352081686668));
#11130=CARTESIAN_POINT('Ctrl Pts',(0.722929908501543,-0.244251601209411,
0.663382628119203));
#11131=CARTESIAN_POINT('Ctrl Pts',(0.750785745543687,-0.232861760990032,
0.631684198665439));
#11132=CARTESIAN_POINT('Ctrl Pts',(0.763642258217232,-0.224161999508995,
0.615966552324775));
#11133=CARTESIAN_POINT('Ctrl Pts',(0.78555112003688,-0.203463743702801,
0.587792702767295));
#11134=CARTESIAN_POINT('Ctrl Pts',(0.795684265985088,-0.190326085855194,
0.573915184558108));
#11135=CARTESIAN_POINT('Ctrl Pts',(0.813159949759,-0.15976606450048,0.548874290046456));
#11136=CARTESIAN_POINT('Ctrl Pts',(0.820511285096538,-0.142345102874864,
0.537715343527944));
#11137=CARTESIAN_POINT('Ctrl Pts',(0.833661031856294,-0.099930567888331,
0.517157748491653));
#11138=CARTESIAN_POINT('Ctrl Pts',(0.838633903678357,-0.0740444353928835,
0.508899795931835));
#11139=CARTESIAN_POINT('Ctrl Pts',(0.841298510752801,-0.0476299999999999,
0.504455939115715));
#11140=CARTESIAN_POINT('',(0.528110872004958,-0.04763,0.871530771444223));
#11141=CARTESIAN_POINT('Origin',(0.707106781186547,-0.04763,0.707106781186548));
#11142=CARTESIAN_POINT('',(0.871530771444223,-0.04763,0.528110872004959));
#11143=CARTESIAN_POINT('Ctrl Pts',(0.871530771444223,-0.0476300000000001,
0.528110872004958));
#11144=CARTESIAN_POINT('Ctrl Pts',(0.87014664509073,-0.0609922781173483,
0.530395067942936));
#11145=CARTESIAN_POINT('Ctrl Pts',(0.868149331745851,-0.0742967091364493,
0.533674141594226));
#11146=CARTESIAN_POINT('Ctrl Pts',(0.85981294420286,-0.115492077056649,
0.54708917182331));
#11147=CARTESIAN_POINT('Ctrl Pts',(0.850993704737257,-0.141695629206859,
0.560922177770136));
#11148=CARTESIAN_POINT('Ctrl Pts',(0.830754510485543,-0.181890537957859,
0.590422647829571));
#11149=CARTESIAN_POINT('Ctrl Pts',(0.816896541396381,-0.201072148666545,
0.609616703125488));
#11150=CARTESIAN_POINT('Ctrl Pts',(0.792310597819928,-0.223955109275652,
0.641117951819998));
#11151=CARTESIAN_POINT('Ctrl Pts',(0.779109323683612,-0.232742381310829,
0.657208095763053));
#11152=CARTESIAN_POINT('Ctrl Pts',(0.750552691816206,-0.244234834628584,
0.68964083160521));
#11153=CARTESIAN_POINT('Ctrl Pts',(0.735185187071673,-0.246942143572133,
0.705971972091755));
#11154=CARTESIAN_POINT('Ctrl Pts',(0.705971972091754,-0.246942143572133,
0.735185187071673));
#11155=CARTESIAN_POINT('Ctrl Pts',(0.689640831605209,-0.244234834628584,
0.750552691816206));
#11156=CARTESIAN_POINT('Ctrl Pts',(0.657208095763052,-0.232742381310829,
0.779109323683612));
#11157=CARTESIAN_POINT('Ctrl Pts',(0.641117951819998,-0.223955109275652,
0.792310597819928));
#11158=CARTESIAN_POINT('Ctrl Pts',(0.609616703125487,-0.201072148666545,
0.816896541396382));
#11159=CARTESIAN_POINT('Ctrl Pts',(0.590422647829571,-0.181890537957858,
0.830754510485544));
#11160=CARTESIAN_POINT('Ctrl Pts',(0.560922177770135,-0.141695629206858,
0.850993704737257));
#11161=CARTESIAN_POINT('Ctrl Pts',(0.547089171823309,-0.115492077056649,
0.859812944202861));
#11162=CARTESIAN_POINT('Ctrl Pts',(0.533674141594226,-0.0742967091364491,
0.868149331745852));
#11163=CARTESIAN_POINT('Ctrl Pts',(0.530395067942936,-0.0609922781173483,
0.870146645090731));
#11164=CARTESIAN_POINT('Ctrl Pts',(0.528110872004958,-0.0476300000000001,
0.871530771444223));
#11165=CARTESIAN_POINT('Origin',(0.707106781186547,-0.04763,0.707106781186548));
#11166=CARTESIAN_POINT('Origin',(0.,-0.166705,0.));
#11167=CARTESIAN_POINT('',(0.242834539687906,-0.04763,0.989696097314));
#11168=CARTESIAN_POINT('Origin',(0.,-0.04763,0.));
#11169=CARTESIAN_POINT('',(-0.242834539687907,-0.04763,0.989696097314));
#11170=CARTESIAN_POINT('Ctrl Pts',(0.242834539687906,-0.04763,0.989696097314));
#11171=CARTESIAN_POINT('Ctrl Pts',(0.24024064412003,-0.0609922781173483,
0.990332542620729));
#11172=CARTESIAN_POINT('Ctrl Pts',(0.236509675094874,-0.0742967091364492,
0.991238884025248));
#11173=CARTESIAN_POINT('Ctrl Pts',(0.221129100087819,-0.115492077056649,
0.994830026707808));
#11174=CARTESIAN_POINT('Ctrl Pts',(0.205111543747588,-0.141695629206859,
0.998375294985966));
#11175=CARTESIAN_POINT('Ctrl Pts',(0.169940289819232,-0.181890537957859,
1.00492400591205));
#11176=CARTESIAN_POINT('Ctrl Pts',(0.1465689792446,-0.201072148666545,1.00869718865384));
#11177=CARTESIAN_POINT('Ctrl Pts',(0.106909345252087,-0.223955109275652,
1.01358704779679));
#11178=CARTESIAN_POINT('Ctrl Pts',(0.0861971848975941,-0.232742381310829,
1.0156297872271));
#11179=CARTESIAN_POINT('Ctrl Pts',(0.0430711894098822,-0.244234834628584,
1.01837060663223));
#11180=CARTESIAN_POINT('Ctrl Pts',(0.0206568624125605,-0.246942143572133,
1.019052));
#11181=CARTESIAN_POINT('Ctrl Pts',(-0.0206568624125608,-0.246942143572133,
1.019052));
#11182=CARTESIAN_POINT('Ctrl Pts',(-0.0430711894098825,-0.244234834628584,
1.01837060663223));
#11183=CARTESIAN_POINT('Ctrl Pts',(-0.0861971848975943,-0.232742381310829,
1.0156297872271));
#11184=CARTESIAN_POINT('Ctrl Pts',(-0.106909345252088,-0.223955109275652,
1.01358704779679));
#11185=CARTESIAN_POINT('Ctrl Pts',(-0.1465689792446,-0.201072148666545,
1.00869718865384));
#11186=CARTESIAN_POINT('Ctrl Pts',(-0.169940289819232,-0.181890537957859,
1.00492400591205));
#11187=CARTESIAN_POINT('Ctrl Pts',(-0.205111543747588,-0.141695629206859,
0.998375294985966));
#11188=CARTESIAN_POINT('Ctrl Pts',(-0.221129100087819,-0.115492077056649,
0.994830026707808));
#11189=CARTESIAN_POINT('Ctrl Pts',(-0.236509675094875,-0.0742967091364493,
0.991238884025248));
#11190=CARTESIAN_POINT('Ctrl Pts',(-0.24024064412003,-0.0609922781173483,
0.990332542620729));
#11191=CARTESIAN_POINT('Ctrl Pts',(-0.242834539687907,-0.04763,0.989696097314));
#11192=CARTESIAN_POINT('',(-0.528110872004959,-0.04763,0.871530771444223));
#11193=CARTESIAN_POINT('Origin',(0.,-0.04763,0.));
#11194=CARTESIAN_POINT('',(-0.871530771444223,-0.04763,0.528110872004958));
#11195=CARTESIAN_POINT('Ctrl Pts',(-0.528110872004958,-0.0476300000000001,
0.871530771444223));
#11196=CARTESIAN_POINT('Ctrl Pts',(-0.530395067942936,-0.0609922781173484,
0.87014664509073));
#11197=CARTESIAN_POINT('Ctrl Pts',(-0.533674141594226,-0.0742967091364493,
0.868149331745851));
#11198=CARTESIAN_POINT('Ctrl Pts',(-0.54708917182331,-0.115492077056649,
0.85981294420286));
#11199=CARTESIAN_POINT('Ctrl Pts',(-0.560922177770136,-0.141695629206859,
0.850993704737257));
#11200=CARTESIAN_POINT('Ctrl Pts',(-0.590422647829571,-0.181890537957859,
0.830754510485543));
#11201=CARTESIAN_POINT('Ctrl Pts',(-0.609616703125488,-0.201072148666545,
0.816896541396381));
#11202=CARTESIAN_POINT('Ctrl Pts',(-0.641117951819998,-0.223955109275652,
0.792310597819928));
#11203=CARTESIAN_POINT('Ctrl Pts',(-0.657208095763053,-0.232742381310829,
0.779109323683611));
#11204=CARTESIAN_POINT('Ctrl Pts',(-0.68964083160521,-0.244234834628584,
0.750552691816205));
#11205=CARTESIAN_POINT('Ctrl Pts',(-0.705971972091755,-0.246942143572133,
0.735185187071673));
#11206=CARTESIAN_POINT('Ctrl Pts',(-0.735185187071673,-0.246942143572133,
0.705971972091754));
#11207=CARTESIAN_POINT('Ctrl Pts',(-0.750552691816206,-0.244234834628584,
0.689640831605209));
#11208=CARTESIAN_POINT('Ctrl Pts',(-0.779109323683612,-0.232742381310829,
0.657208095763052));
#11209=CARTESIAN_POINT('Ctrl Pts',(-0.792310597819928,-0.223955109275652,
0.641117951819998));
#11210=CARTESIAN_POINT('Ctrl Pts',(-0.816896541396382,-0.201072148666545,
0.609616703125487));
#11211=CARTESIAN_POINT('Ctrl Pts',(-0.830754510485544,-0.181890537957858,
0.590422647829571));
#11212=CARTESIAN_POINT('Ctrl Pts',(-0.850993704737257,-0.141695629206858,
0.560922177770135));
#11213=CARTESIAN_POINT('Ctrl Pts',(-0.859812944202861,-0.115492077056649,
0.547089171823309));
#11214=CARTESIAN_POINT('Ctrl Pts',(-0.868149331745852,-0.0742967091364491,
0.533674141594226));
#11215=CARTESIAN_POINT('Ctrl Pts',(-0.870146645090731,-0.0609922781173483,
0.530395067942936));
#11216=CARTESIAN_POINT('Ctrl Pts',(-0.871530771444223,-0.04763,0.528110872004958));
#11217=CARTESIAN_POINT('',(-0.989696097314,-0.04763,0.242834539687906));
#11218=CARTESIAN_POINT('Origin',(0.,-0.04763,0.));
#11219=CARTESIAN_POINT('',(-1.019052,-0.246942143572133,1.248489836334E-16));
#11220=CARTESIAN_POINT('Ctrl Pts',(-0.989696097314,-0.04763,0.242834539687906));
#11221=CARTESIAN_POINT('Ctrl Pts',(-0.990332542620729,-0.0609922781173483,
0.24024064412003));
#11222=CARTESIAN_POINT('Ctrl Pts',(-0.991238884025248,-0.0742967091364492,
0.236509675094874));
#11223=CARTESIAN_POINT('Ctrl Pts',(-0.994830026707808,-0.115492077056649,
0.221129100087819));
#11224=CARTESIAN_POINT('Ctrl Pts',(-0.998375294985966,-0.141695629206859,
0.205111543747588));
#11225=CARTESIAN_POINT('Ctrl Pts',(-1.00492400591205,-0.181890537957859,
0.169940289819232));
#11226=CARTESIAN_POINT('Ctrl Pts',(-1.00869718865384,-0.201072148666545,
0.1465689792446));
#11227=CARTESIAN_POINT('Ctrl Pts',(-1.01358704779679,-0.223955109275652,
0.106909345252088));
#11228=CARTESIAN_POINT('Ctrl Pts',(-1.0156297872271,-0.232742381310829,
0.0861971848975944));
#11229=CARTESIAN_POINT('Ctrl Pts',(-1.01837060663223,-0.244234834628584,
0.0430711894098825));
#11230=CARTESIAN_POINT('Ctrl Pts',(-1.019052,-0.246942143572133,0.0206568624125608));
#11231=CARTESIAN_POINT('Ctrl Pts',(-1.019052,-0.246942143572133,1.2490009027033E-16));
#11232=CARTESIAN_POINT('',(-1.019052,-0.28578,1.24797876996471E-16));
#11233=CARTESIAN_POINT('',(-1.019052,-0.166705,1.24797876996471E-16));
#11234=CARTESIAN_POINT('Origin',(0.,-0.28578,0.));
#11235=CARTESIAN_POINT('',(-0.989696097314,-0.04763,-0.242834539687906));
#11236=CARTESIAN_POINT('Ctrl Pts',(-1.019052,-0.246942143572133,1.2490009027033E-16));
#11237=CARTESIAN_POINT('Ctrl Pts',(-1.019052,-0.246942143572133,-0.0206568624125605));
#11238=CARTESIAN_POINT('Ctrl Pts',(-1.01837060663223,-0.244234834628584,
-0.0430711894098822));
#11239=CARTESIAN_POINT('Ctrl Pts',(-1.0156297872271,-0.232742381310829,
-0.0861971848975941));
#11240=CARTESIAN_POINT('Ctrl Pts',(-1.01358704779679,-0.223955109275652,
-0.106909345252087));
#11241=CARTESIAN_POINT('Ctrl Pts',(-1.00869718865384,-0.201072148666546,
-0.1465689792446));
#11242=CARTESIAN_POINT('Ctrl Pts',(-1.00492400591205,-0.181890537957859,
-0.169940289819232));
#11243=CARTESIAN_POINT('Ctrl Pts',(-0.998375294985966,-0.141695629206859,
-0.205111543747588));
#11244=CARTESIAN_POINT('Ctrl Pts',(-0.994830026707808,-0.11549207705665,
-0.221129100087819));
#11245=CARTESIAN_POINT('Ctrl Pts',(-0.991238884025248,-0.0742967091364495,
-0.236509675094874));
#11246=CARTESIAN_POINT('Ctrl Pts',(-0.990332542620729,-0.0609922781173484,
-0.24024064412003));
#11247=CARTESIAN_POINT('Ctrl Pts',(-0.989696097314,-0.0476300000000001,
-0.242834539687907));
#11248=CARTESIAN_POINT('',(-0.871530771444223,-0.04763,-0.528110872004958));
#11249=CARTESIAN_POINT('Origin',(0.,-0.04763,0.));
#11250=CARTESIAN_POINT('',(-0.528110872004958,-0.04763,-0.871530771444223));
#11251=CARTESIAN_POINT('Ctrl Pts',(-0.871530771444223,-0.0476300000000001,
-0.528110872004958));
#11252=CARTESIAN_POINT('Ctrl Pts',(-0.87014664509073,-0.0609922781173484,
-0.530395067942936));
#11253=CARTESIAN_POINT('Ctrl Pts',(-0.868149331745851,-0.0742967091364494,
-0.533674141594226));
#11254=CARTESIAN_POINT('Ctrl Pts',(-0.85981294420286,-0.115492077056649,
-0.54708917182331));
#11255=CARTESIAN_POINT('Ctrl Pts',(-0.850993704737257,-0.141695629206859,
-0.560922177770136));
#11256=CARTESIAN_POINT('Ctrl Pts',(-0.830754510485543,-0.181890537957859,
-0.590422647829571));
#11257=CARTESIAN_POINT('Ctrl Pts',(-0.816896541396381,-0.201072148666546,
-0.609616703125488));
#11258=CARTESIAN_POINT('Ctrl Pts',(-0.792310597819928,-0.223955109275652,
-0.641117951819999));
#11259=CARTESIAN_POINT('Ctrl Pts',(-0.779109323683611,-0.232742381310829,
-0.657208095763053));
#11260=CARTESIAN_POINT('Ctrl Pts',(-0.750552691816205,-0.244234834628584,
-0.68964083160521));
#11261=CARTESIAN_POINT('Ctrl Pts',(-0.735185187071673,-0.246942143572133,
-0.705971972091755));
#11262=CARTESIAN_POINT('Ctrl Pts',(-0.705971972091754,-0.246942143572133,
-0.735185187071673));
#11263=CARTESIAN_POINT('Ctrl Pts',(-0.68964083160521,-0.244234834628584,
-0.750552691816206));
#11264=CARTESIAN_POINT('Ctrl Pts',(-0.657208095763052,-0.232742381310829,
-0.779109323683612));
#11265=CARTESIAN_POINT('Ctrl Pts',(-0.641117951819998,-0.223955109275652,
-0.792310597819928));
#11266=CARTESIAN_POINT('Ctrl Pts',(-0.609616703125488,-0.201072148666545,
-0.816896541396381));
#11267=CARTESIAN_POINT('Ctrl Pts',(-0.590422647829571,-0.181890537957859,
-0.830754510485543));
#11268=CARTESIAN_POINT('Ctrl Pts',(-0.560922177770136,-0.141695629206859,
-0.850993704737257));
#11269=CARTESIAN_POINT('Ctrl Pts',(-0.54708917182331,-0.115492077056649,
-0.85981294420286));
#11270=CARTESIAN_POINT('Ctrl Pts',(-0.533674141594226,-0.0742967091364494,
-0.868149331745852));
#11271=CARTESIAN_POINT('Ctrl Pts',(-0.530395067942936,-0.0609922781173484,
-0.870146645090731));
#11272=CARTESIAN_POINT('Ctrl Pts',(-0.528110872004958,-0.0476300000000001,
-0.871530771444223));
#11273=CARTESIAN_POINT('',(-0.242834539687906,-0.04763,-0.989696097314));
#11274=CARTESIAN_POINT('Origin',(0.,-0.04763,0.));
#11275=CARTESIAN_POINT('',(0.242834539687906,-0.04763,-0.989696097314));
#11276=CARTESIAN_POINT('Ctrl Pts',(-0.242834539687907,-0.04763,-0.989696097314));
#11277=CARTESIAN_POINT('Ctrl Pts',(-0.24024064412003,-0.0609922781173483,
-0.990332542620729));
#11278=CARTESIAN_POINT('Ctrl Pts',(-0.236509675094874,-0.0742967091364493,
-0.991238884025248));
#11279=CARTESIAN_POINT('Ctrl Pts',(-0.221129100087819,-0.115492077056649,
-0.994830026707808));
#11280=CARTESIAN_POINT('Ctrl Pts',(-0.205111543747588,-0.141695629206859,
-0.998375294985966));
#11281=CARTESIAN_POINT('Ctrl Pts',(-0.169940289819232,-0.181890537957859,
-1.00492400591205));
#11282=CARTESIAN_POINT('Ctrl Pts',(-0.1465689792446,-0.201072148666545,
-1.00869718865384));
#11283=CARTESIAN_POINT('Ctrl Pts',(-0.106909345252087,-0.223955109275652,
-1.01358704779679));
#11284=CARTESIAN_POINT('Ctrl Pts',(-0.0861971848975942,-0.232742381310829,
-1.0156297872271));
#11285=CARTESIAN_POINT('Ctrl Pts',(-0.0430711894098823,-0.244234834628584,
-1.01837060663223));
#11286=CARTESIAN_POINT('Ctrl Pts',(-0.0206568624125606,-0.246942143572133,
-1.019052));
#11287=CARTESIAN_POINT('Ctrl Pts',(0.0206568624125607,-0.246942143572133,
-1.019052));
#11288=CARTESIAN_POINT('Ctrl Pts',(0.0430711894098824,-0.244234834628584,
-1.01837060663223));
#11289=CARTESIAN_POINT('Ctrl Pts',(0.0861971848975943,-0.232742381310829,
-1.0156297872271));
#11290=CARTESIAN_POINT('Ctrl Pts',(0.106909345252088,-0.223955109275652,
-1.01358704779679));
#11291=CARTESIAN_POINT('Ctrl Pts',(0.1465689792446,-0.201072148666545,-1.00869718865384));
#11292=CARTESIAN_POINT('Ctrl Pts',(0.169940289819232,-0.181890537957859,
-1.00492400591205));
#11293=CARTESIAN_POINT('Ctrl Pts',(0.205111543747588,-0.141695629206859,
-0.998375294985966));
#11294=CARTESIAN_POINT('Ctrl Pts',(0.221129100087819,-0.115492077056649,
-0.994830026707808));
#11295=CARTESIAN_POINT('Ctrl Pts',(0.236509675094874,-0.0742967091364493,
-0.991238884025248));
#11296=CARTESIAN_POINT('Ctrl Pts',(0.24024064412003,-0.0609922781173484,
-0.990332542620729));
#11297=CARTESIAN_POINT('Ctrl Pts',(0.242834539687907,-0.04763,-0.989696097314));
#11298=CARTESIAN_POINT('',(0.528110872004958,-0.04763,-0.871530771444223));
#11299=CARTESIAN_POINT('Origin',(0.,-0.04763,0.));
#11300=CARTESIAN_POINT('',(0.871530771444223,-0.04763,-0.528110872004958));
#11301=CARTESIAN_POINT('Ctrl Pts',(0.528110872004958,-0.0476300000000001,
-0.871530771444223));
#11302=CARTESIAN_POINT('Ctrl Pts',(0.530395067942936,-0.0609922781173484,
-0.870146645090731));
#11303=CARTESIAN_POINT('Ctrl Pts',(0.533674141594226,-0.0742967091364493,
-0.868149331745851));
#11304=CARTESIAN_POINT('Ctrl Pts',(0.54708917182331,-0.115492077056649,
-0.85981294420286));
#11305=CARTESIAN_POINT('Ctrl Pts',(0.560922177770136,-0.141695629206859,
-0.850993704737257));
#11306=CARTESIAN_POINT('Ctrl Pts',(0.590422647829571,-0.181890537957859,
-0.830754510485543));
#11307=CARTESIAN_POINT('Ctrl Pts',(0.609616703125488,-0.201072148666545,
-0.816896541396381));
#11308=CARTESIAN_POINT('Ctrl Pts',(0.641117951819998,-0.223955109275652,
-0.792310597819928));
#11309=CARTESIAN_POINT('Ctrl Pts',(0.657208095763053,-0.232742381310829,
-0.779109323683612));
#11310=CARTESIAN_POINT('Ctrl Pts',(0.68964083160521,-0.244234834628584,
-0.750552691816206));
#11311=CARTESIAN_POINT('Ctrl Pts',(0.705971972091755,-0.246942143572133,
-0.735185187071673));
#11312=CARTESIAN_POINT('Ctrl Pts',(0.735185187071673,-0.246942143572133,
-0.705971972091754));
#11313=CARTESIAN_POINT('Ctrl Pts',(0.750552691816206,-0.244234834628584,
-0.68964083160521));
#11314=CARTESIAN_POINT('Ctrl Pts',(0.779109323683612,-0.232742381310829,
-0.657208095763053));
#11315=CARTESIAN_POINT('Ctrl Pts',(0.792310597819928,-0.223955109275652,
-0.641117951819998));
#11316=CARTESIAN_POINT('Ctrl Pts',(0.816896541396381,-0.201072148666545,
-0.609616703125488));
#11317=CARTESIAN_POINT('Ctrl Pts',(0.830754510485543,-0.181890537957859,
-0.590422647829571));
#11318=CARTESIAN_POINT('Ctrl Pts',(0.850993704737257,-0.141695629206859,
-0.560922177770136));
#11319=CARTESIAN_POINT('Ctrl Pts',(0.85981294420286,-0.115492077056649,
-0.54708917182331));
#11320=CARTESIAN_POINT('Ctrl Pts',(0.868149331745851,-0.0742967091364493,
-0.533674141594226));
#11321=CARTESIAN_POINT('Ctrl Pts',(0.870146645090731,-0.0609922781173484,
-0.530395067942936));
#11322=CARTESIAN_POINT('Ctrl Pts',(0.871530771444223,-0.0476300000000001,
-0.528110872004958));
#11323=CARTESIAN_POINT('',(0.989696097314,-0.04763,-0.242834539687906));
#11324=CARTESIAN_POINT('Origin',(0.,-0.04763,0.));
#11325=CARTESIAN_POINT('',(0.989696097314,-0.04763,0.242834539687906));
#11326=CARTESIAN_POINT('Ctrl Pts',(0.989696097314,-0.04763,-0.242834539687907));
#11327=CARTESIAN_POINT('Ctrl Pts',(0.990332542620729,-0.0609922781173483,
-0.24024064412003));
#11328=CARTESIAN_POINT('Ctrl Pts',(0.991238884025248,-0.0742967091364493,
-0.236509675094874));
#11329=CARTESIAN_POINT('Ctrl Pts',(0.994830026707808,-0.115492077056649,
-0.221129100087819));
#11330=CARTESIAN_POINT('Ctrl Pts',(0.998375294985966,-0.141695629206859,
-0.205111543747588));
#11331=CARTESIAN_POINT('Ctrl Pts',(1.00492400591205,-0.181890537957859,
-0.169940289819232));
#11332=CARTESIAN_POINT('Ctrl Pts',(1.00869718865384,-0.201072148666545,
-0.1465689792446));
#11333=CARTESIAN_POINT('Ctrl Pts',(1.01358704779679,-0.223955109275652,
-0.106909345252087));
#11334=CARTESIAN_POINT('Ctrl Pts',(1.0156297872271,-0.232742381310829,-0.0861971848975942));
#11335=CARTESIAN_POINT('Ctrl Pts',(1.01837060663223,-0.244234834628584,
-0.0430711894098823));
#11336=CARTESIAN_POINT('Ctrl Pts',(1.019052,-0.246942143572133,-0.0206568624125607));
#11337=CARTESIAN_POINT('Ctrl Pts',(1.019052,-0.246942143572133,0.0206568624125607));
#11338=CARTESIAN_POINT('Ctrl Pts',(1.01837060663223,-0.244234834628584,
0.0430711894098823));
#11339=CARTESIAN_POINT('Ctrl Pts',(1.0156297872271,-0.232742381310829,0.0861971848975942));
#11340=CARTESIAN_POINT('Ctrl Pts',(1.01358704779679,-0.223955109275652,
0.106909345252087));
#11341=CARTESIAN_POINT('Ctrl Pts',(1.00869718865384,-0.201072148666545,
0.1465689792446));
#11342=CARTESIAN_POINT('Ctrl Pts',(1.00492400591205,-0.181890537957859,
0.169940289819232));
#11343=CARTESIAN_POINT('Ctrl Pts',(0.998375294985966,-0.141695629206859,
0.205111543747588));
#11344=CARTESIAN_POINT('Ctrl Pts',(0.994830026707808,-0.115492077056649,
0.221129100087819));
#11345=CARTESIAN_POINT('Ctrl Pts',(0.991238884025248,-0.0742967091364492,
0.236509675094874));
#11346=CARTESIAN_POINT('Ctrl Pts',(0.990332542620729,-0.0609922781173483,
0.24024064412003));
#11347=CARTESIAN_POINT('Ctrl Pts',(0.989696097314,-0.04763,0.242834539687907));
#11348=CARTESIAN_POINT('Origin',(0.,-0.04763,0.));
#11349=CARTESIAN_POINT('Origin',(0.,-0.04763,0.));
#11350=CARTESIAN_POINT('',(0.238183666596899,-0.04763,0.951592097314));
#11351=CARTESIAN_POINT('Origin',(0.,-0.04763,0.));
#11352=CARTESIAN_POINT('Origin',(-1.94289029309402E-16,-0.04763,1.));
#11353=CARTESIAN_POINT('Origin',(-1.94289029309402E-16,0.,1.));
#11354=CARTESIAN_POINT('',(-0.2381836665969,-0.04763,0.951592097314));
#11355=CARTESIAN_POINT('Ctrl Pts',(-0.238183666596899,-0.0476299999999999,
0.951592097314));
#11356=CARTESIAN_POINT('Ctrl Pts',(-0.233157223576062,-0.0740444353928835,
0.952850216871763));
#11357=CARTESIAN_POINT('Ctrl Pts',(-0.223801617934946,-0.0999305678883309,
0.955173119738174));
#11358=CARTESIAN_POINT('Ctrl Pts',(-0.199966927975188,-0.142345102874864,
0.960411259488514));
#11359=CARTESIAN_POINT('Ctrl Pts',(-0.1868781821531,-0.159766064500479,
0.963103647174702));
#11360=CARTESIAN_POINT('Ctrl Pts',(-0.15681442133453,-0.190326085855194,
0.968453058988463));
#11361=CARTESIAN_POINT('Ctrl Pts',(-0.139836317888043,-0.203463743702801,
0.971100730005489));
#11362=CARTESIAN_POINT('Ctrl Pts',(-0.104422493053067,-0.224161999508995,
0.975530745318961));
#11363=CARTESIAN_POINT('Ctrl Pts',(-0.0842175114474176,-0.232861760990032,
0.977553872336861));
#11364=CARTESIAN_POINT('Ctrl Pts',(-0.0421062857595701,-0.244251601209411,
0.980270995488453));
#11365=CARTESIAN_POINT('Ctrl Pts',(-0.0201990724523197,-0.246942143572133,
0.980948));
#11366=CARTESIAN_POINT('Ctrl Pts',(0.020199072452319,-0.246942143572133,
0.980948));
#11367=CARTESIAN_POINT('Ctrl Pts',(0.0421062857595694,-0.244251601209411,
0.980270995488454));
#11368=CARTESIAN_POINT('Ctrl Pts',(0.0842175114474169,-0.232861760990032,
0.977553872336861));
#11369=CARTESIAN_POINT('Ctrl Pts',(0.104422493053067,-0.224161999508995,
0.975530745318961));
#11370=CARTESIAN_POINT('Ctrl Pts',(0.139836317888042,-0.203463743702801,
0.971100730005489));
#11371=CARTESIAN_POINT('Ctrl Pts',(0.15681442133453,-0.190326085855194,
0.968453058988463));
#11372=CARTESIAN_POINT('Ctrl Pts',(0.1868781821531,-0.15976606450048,0.963103647174702));
#11373=CARTESIAN_POINT('Ctrl Pts',(0.199966927975188,-0.142345102874864,
0.960411259488514));
#11374=CARTESIAN_POINT('Ctrl Pts',(0.223801617934945,-0.0999305678883309,
0.955173119738174));
#11375=CARTESIAN_POINT('Ctrl Pts',(0.233157223576061,-0.0740444353928835,
0.952850216871763));
#11376=CARTESIAN_POINT('Ctrl Pts',(0.238183666596899,-0.0476299999999999,
0.951592097314));
#11377=CARTESIAN_POINT('Origin',(-1.94289029309402E-16,-0.04763,1.));
#11378=CARTESIAN_POINT('Origin',(0.,-0.04763,0.));
#11379=CARTESIAN_POINT('',(-0.504455939115715,-0.04763,0.841298510752802));
#11380=CARTESIAN_POINT('Origin',(0.,-0.04763,0.));
#11381=CARTESIAN_POINT('Origin',(-0.707106781186548,-0.04763,0.707106781186547));
#11382=CARTESIAN_POINT('Origin',(-0.707106781186548,0.,0.707106781186547));
#11383=CARTESIAN_POINT('',(-0.841298510752802,-0.04763,0.504455939115715));
#11384=CARTESIAN_POINT('Ctrl Pts',(-0.841298510752802,-0.04763,0.504455939115715));
#11385=CARTESIAN_POINT('Ctrl Pts',(-0.838633903678357,-0.0740444353928835,
0.508899795931835));
#11386=CARTESIAN_POINT('Ctrl Pts',(-0.833661031856294,-0.0999305678883309,
0.517157748491652));
#11387=CARTESIAN_POINT('Ctrl Pts',(-0.820511285096538,-0.142345102874864,
0.537715343527944));
#11388=CARTESIAN_POINT('Ctrl Pts',(-0.813159949759,-0.159766064500479,0.548874290046456));
#11389=CARTESIAN_POINT('Ctrl Pts',(-0.795684265985089,-0.190326085855194,
0.573915184558107));
#11390=CARTESIAN_POINT('Ctrl Pts',(-0.78555112003688,-0.203463743702801,
0.587792702767295));
#11391=CARTESIAN_POINT('Ctrl Pts',(-0.763642258217233,-0.224161999508995,
0.615966552324775));
#11392=CARTESIAN_POINT('Ctrl Pts',(-0.750785745543687,-0.232861760990032,
0.631684198665438));
#11393=CARTESIAN_POINT('Ctrl Pts',(-0.722929908501543,-0.244251601209411,
0.663382628119203));
#11394=CARTESIAN_POINT('Ctrl Pts',(-0.707917883896095,-0.246942143572133,
0.679352081686668));
#11395=CARTESIAN_POINT('Ctrl Pts',(-0.679352081686668,-0.246942143572133,
0.707917883896095));
#11396=CARTESIAN_POINT('Ctrl Pts',(-0.663382628119203,-0.244251601209411,
0.722929908501544));
#11397=CARTESIAN_POINT('Ctrl Pts',(-0.631684198665438,-0.232861760990031,
0.750785745543687));
#11398=CARTESIAN_POINT('Ctrl Pts',(-0.615966552324775,-0.224161999508995,
0.763642258217233));
#11399=CARTESIAN_POINT('Ctrl Pts',(-0.587792702767295,-0.203463743702801,
0.78555112003688));
#11400=CARTESIAN_POINT('Ctrl Pts',(-0.573915184558107,-0.190326085855194,
0.795684265985088));
#11401=CARTESIAN_POINT('Ctrl Pts',(-0.548874290046456,-0.159766064500479,
0.813159949759));
#11402=CARTESIAN_POINT('Ctrl Pts',(-0.537715343527944,-0.142345102874864,
0.820511285096538));
#11403=CARTESIAN_POINT('Ctrl Pts',(-0.517157748491652,-0.0999305678883309,
0.833661031856294));
#11404=CARTESIAN_POINT('Ctrl Pts',(-0.508899795931835,-0.0740444353928835,
0.838633903678357));
#11405=CARTESIAN_POINT('Ctrl Pts',(-0.504455939115716,-0.04763,0.841298510752801));
#11406=CARTESIAN_POINT('Origin',(-0.707106781186548,-0.04763,0.707106781186547));
#11407=CARTESIAN_POINT('Origin',(0.,-0.04763,0.));
#11408=CARTESIAN_POINT('',(-0.951592097314,-0.04763,0.238183666596899));
#11409=CARTESIAN_POINT('Origin',(0.,-0.04763,0.));
#11410=CARTESIAN_POINT('Origin',(-1.,-0.04763,-1.11022302462516E-16));
#11411=CARTESIAN_POINT('Origin',(-1.,0.,-1.11022302462516E-16));
#11412=CARTESIAN_POINT('',(-0.951592097314,-0.04763,-0.2381836665969));
#11413=CARTESIAN_POINT('',(-0.980948,-0.246942143572133,1.08514323328844E-18));
#11414=CARTESIAN_POINT('Ctrl Pts',(-0.951592097314,-0.04763,-0.238183666596899));
#11415=CARTESIAN_POINT('Ctrl Pts',(-0.952850216871763,-0.0740444353928835,
-0.233157223576062));
#11416=CARTESIAN_POINT('Ctrl Pts',(-0.955173119738174,-0.0999305678883309,
-0.223801617934946));
#11417=CARTESIAN_POINT('Ctrl Pts',(-0.960411259488514,-0.142345102874864,
-0.199966927975188));
#11418=CARTESIAN_POINT('Ctrl Pts',(-0.963103647174702,-0.159766064500479,
-0.1868781821531));
#11419=CARTESIAN_POINT('Ctrl Pts',(-0.968453058988463,-0.190326085855194,
-0.15681442133453));
#11420=CARTESIAN_POINT('Ctrl Pts',(-0.971100730005489,-0.203463743702801,
-0.139836317888043));
#11421=CARTESIAN_POINT('Ctrl Pts',(-0.975530745318961,-0.224161999508995,
-0.104422493053067));
#11422=CARTESIAN_POINT('Ctrl Pts',(-0.977553872336861,-0.232861760990032,
-0.0842175114474175));
#11423=CARTESIAN_POINT('Ctrl Pts',(-0.980270995488453,-0.244251601209411,
-0.0421062857595699));
#11424=CARTESIAN_POINT('Ctrl Pts',(-0.980948,-0.246942143572133,-0.0201990724523195));
#11425=CARTESIAN_POINT('Ctrl Pts',(-0.980948,-0.246942143572133,-1.17961196366423E-16));
#11426=CARTESIAN_POINT('Origin',(-1.,-0.04763,-1.11022302462516E-16));
#11427=CARTESIAN_POINT('Ctrl Pts',(-0.980948,-0.246942143572133,-1.17961196366423E-16));
#11428=CARTESIAN_POINT('Ctrl Pts',(-0.980948,-0.246942143572133,0.0201990724523192));
#11429=CARTESIAN_POINT('Ctrl Pts',(-0.980270995488453,-0.244251601209411,
0.0421062857595695));
#11430=CARTESIAN_POINT('Ctrl Pts',(-0.977553872336861,-0.232861760990032,
0.0842175114474169));
#11431=CARTESIAN_POINT('Ctrl Pts',(-0.975530745318961,-0.224161999508995,
0.104422493053066));
#11432=CARTESIAN_POINT('Ctrl Pts',(-0.971100730005489,-0.203463743702801,
0.139836317888042));
#11433=CARTESIAN_POINT('Ctrl Pts',(-0.968453058988463,-0.190326085855194,
0.15681442133453));
#11434=CARTESIAN_POINT('Ctrl Pts',(-0.963103647174702,-0.15976606450048,
0.1868781821531));
#11435=CARTESIAN_POINT('Ctrl Pts',(-0.960411259488514,-0.142345102874864,
0.199966927975188));
#11436=CARTESIAN_POINT('Ctrl Pts',(-0.955173119738174,-0.099930567888331,
0.223801617934945));
#11437=CARTESIAN_POINT('Ctrl Pts',(-0.952850216871763,-0.0740444353928835,
0.233157223576061));
#11438=CARTESIAN_POINT('Ctrl Pts',(-0.951592097314,-0.04763,0.238183666596899));
#11439=CARTESIAN_POINT('Origin',(0.,-0.04763,0.));
#11440=CARTESIAN_POINT('',(-0.841298510752802,-0.04763,-0.504455939115715));
#11441=CARTESIAN_POINT('Origin',(0.,-0.04763,0.));
#11442=CARTESIAN_POINT('Origin',(-0.707106781186547,-0.04763,-0.707106781186548));
#11443=CARTESIAN_POINT('Origin',(-0.707106781186547,0.,-0.707106781186548));
#11444=CARTESIAN_POINT('',(-0.504455939115715,-0.04763,-0.841298510752802));
#11445=CARTESIAN_POINT('Ctrl Pts',(-0.504455939115715,-0.04763,-0.841298510752802));
#11446=CARTESIAN_POINT('Ctrl Pts',(-0.508899795931835,-0.0740444353928835,
-0.838633903678357));
#11447=CARTESIAN_POINT('Ctrl Pts',(-0.517157748491652,-0.0999305678883309,
-0.833661031856294));
#11448=CARTESIAN_POINT('Ctrl Pts',(-0.537715343527944,-0.142345102874864,
-0.820511285096538));
#11449=CARTESIAN_POINT('Ctrl Pts',(-0.548874290046456,-0.159766064500479,
-0.813159949759));
#11450=CARTESIAN_POINT('Ctrl Pts',(-0.573915184558107,-0.190326085855194,
-0.795684265985089));
#11451=CARTESIAN_POINT('Ctrl Pts',(-0.587792702767295,-0.203463743702801,
-0.78555112003688));
#11452=CARTESIAN_POINT('Ctrl Pts',(-0.615966552324775,-0.224161999508995,
-0.763642258217233));
#11453=CARTESIAN_POINT('Ctrl Pts',(-0.631684198665438,-0.232861760990032,
-0.750785745543687));
#11454=CARTESIAN_POINT('Ctrl Pts',(-0.663382628119203,-0.244251601209411,
-0.722929908501543));
#11455=CARTESIAN_POINT('Ctrl Pts',(-0.679352081686668,-0.246942143572133,
-0.707917883896095));
#11456=CARTESIAN_POINT('Ctrl Pts',(-0.707917883896095,-0.246942143572133,
-0.679352081686668));
#11457=CARTESIAN_POINT('Ctrl Pts',(-0.722929908501543,-0.244251601209411,
-0.663382628119203));
#11458=CARTESIAN_POINT('Ctrl Pts',(-0.750785745543687,-0.232861760990032,
-0.631684198665439));
#11459=CARTESIAN_POINT('Ctrl Pts',(-0.763642258217232,-0.224161999508995,
-0.615966552324775));
#11460=CARTESIAN_POINT('Ctrl Pts',(-0.78555112003688,-0.203463743702801,
-0.587792702767295));
#11461=CARTESIAN_POINT('Ctrl Pts',(-0.795684265985088,-0.190326085855194,
-0.573915184558107));
#11462=CARTESIAN_POINT('Ctrl Pts',(-0.813159949759,-0.15976606450048,-0.548874290046456));
#11463=CARTESIAN_POINT('Ctrl Pts',(-0.820511285096538,-0.142345102874864,
-0.537715343527944));
#11464=CARTESIAN_POINT('Ctrl Pts',(-0.833661031856294,-0.0999305678883311,
-0.517157748491652));
#11465=CARTESIAN_POINT('Ctrl Pts',(-0.838633903678357,-0.0740444353928836,
-0.508899795931835));
#11466=CARTESIAN_POINT('Ctrl Pts',(-0.841298510752801,-0.04763,-0.504455939115715));
#11467=CARTESIAN_POINT('Origin',(-0.707106781186547,-0.04763,-0.707106781186548));
#11468=CARTESIAN_POINT('Origin',(0.,-0.04763,0.));
#11469=CARTESIAN_POINT('',(-0.238183666596899,-0.04763,-0.951592097314));
#11470=CARTESIAN_POINT('Origin',(0.,-0.04763,0.));
#11471=CARTESIAN_POINT('Origin',(5.55111512312578E-17,-0.04763,-1.));
#11472=CARTESIAN_POINT('Origin',(5.55111512312578E-17,0.,-1.));
#11473=CARTESIAN_POINT('',(0.238183666596899,-0.04763,-0.951592097314));
#11474=CARTESIAN_POINT('Ctrl Pts',(0.238183666596899,-0.04763,-0.951592097314));
#11475=CARTESIAN_POINT('Ctrl Pts',(0.233157223576062,-0.0740444353928835,
-0.952850216871763));
#11476=CARTESIAN_POINT('Ctrl Pts',(0.223801617934946,-0.099930567888331,
-0.955173119738174));
#11477=CARTESIAN_POINT('Ctrl Pts',(0.199966927975188,-0.142345102874864,
-0.960411259488514));
#11478=CARTESIAN_POINT('Ctrl Pts',(0.1868781821531,-0.15976606450048,-0.963103647174702));
#11479=CARTESIAN_POINT('Ctrl Pts',(0.15681442133453,-0.190326085855194,
-0.968453058988463));
#11480=CARTESIAN_POINT('Ctrl Pts',(0.139836317888042,-0.203463743702801,
-0.971100730005489));
#11481=CARTESIAN_POINT('Ctrl Pts',(0.104422493053067,-0.224161999508995,
-0.975530745318961));
#11482=CARTESIAN_POINT('Ctrl Pts',(0.0842175114474173,-0.232861760990032,
-0.977553872336861));
#11483=CARTESIAN_POINT('Ctrl Pts',(0.0421062857595698,-0.244251601209411,
-0.980270995488453));
#11484=CARTESIAN_POINT('Ctrl Pts',(0.0201990724523194,-0.246942143572133,
-0.980948));
#11485=CARTESIAN_POINT('Ctrl Pts',(-0.0201990724523193,-0.246942143572133,
-0.980948));
#11486=CARTESIAN_POINT('Ctrl Pts',(-0.0421062857595697,-0.244251601209411,
-0.980270995488453));
#11487=CARTESIAN_POINT('Ctrl Pts',(-0.0842175114474171,-0.232861760990032,
-0.977553872336861));
#11488=CARTESIAN_POINT('Ctrl Pts',(-0.104422493053067,-0.224161999508995,
-0.975530745318961));
#11489=CARTESIAN_POINT('Ctrl Pts',(-0.139836317888042,-0.203463743702801,
-0.971100730005489));
#11490=CARTESIAN_POINT('Ctrl Pts',(-0.15681442133453,-0.190326085855194,
-0.968453058988463));
#11491=CARTESIAN_POINT('Ctrl Pts',(-0.1868781821531,-0.15976606450048,-0.963103647174702));
#11492=CARTESIAN_POINT('Ctrl Pts',(-0.199966927975188,-0.142345102874864,
-0.960411259488514));
#11493=CARTESIAN_POINT('Ctrl Pts',(-0.223801617934945,-0.099930567888331,
-0.955173119738174));
#11494=CARTESIAN_POINT('Ctrl Pts',(-0.233157223576062,-0.0740444353928835,
-0.952850216871763));
#11495=CARTESIAN_POINT('Ctrl Pts',(-0.238183666596899,-0.0476299999999999,
-0.951592097314));
#11496=CARTESIAN_POINT('Origin',(5.55111512312578E-17,-0.04763,-1.));
#11497=CARTESIAN_POINT('Origin',(0.,-0.04763,0.));
#11498=CARTESIAN_POINT('',(0.504455939115715,-0.04763,-0.841298510752802));
#11499=CARTESIAN_POINT('Origin',(0.,-0.04763,0.));
#11500=CARTESIAN_POINT('Origin',(0.707106781186548,-0.04763,-0.707106781186547));
#11501=CARTESIAN_POINT('Origin',(0.707106781186548,0.,-0.707106781186547));
#11502=CARTESIAN_POINT('',(0.841298510752802,-0.04763,-0.504455939115715));
#11503=CARTESIAN_POINT('Ctrl Pts',(0.841298510752802,-0.04763,-0.504455939115715));
#11504=CARTESIAN_POINT('Ctrl Pts',(0.838633903678357,-0.0740444353928835,
-0.508899795931835));
#11505=CARTESIAN_POINT('Ctrl Pts',(0.833661031856294,-0.0999305678883309,
-0.517157748491652));
#11506=CARTESIAN_POINT('Ctrl Pts',(0.820511285096538,-0.142345102874864,
-0.537715343527944));
#11507=CARTESIAN_POINT('Ctrl Pts',(0.813159949759,-0.159766064500479,-0.548874290046456));
#11508=CARTESIAN_POINT('Ctrl Pts',(0.795684265985088,-0.190326085855194,
-0.573915184558107));
#11509=CARTESIAN_POINT('Ctrl Pts',(0.78555112003688,-0.203463743702801,
-0.587792702767295));
#11510=CARTESIAN_POINT('Ctrl Pts',(0.763642258217233,-0.224161999508995,
-0.615966552324775));
#11511=CARTESIAN_POINT('Ctrl Pts',(0.750785745543687,-0.232861760990032,
-0.631684198665438));
#11512=CARTESIAN_POINT('Ctrl Pts',(0.722929908501543,-0.244251601209411,
-0.663382628119203));
#11513=CARTESIAN_POINT('Ctrl Pts',(0.707917883896095,-0.246942143572133,
-0.679352081686668));
#11514=CARTESIAN_POINT('Ctrl Pts',(0.679352081686668,-0.246942143572133,
-0.707917883896095));
#11515=CARTESIAN_POINT('Ctrl Pts',(0.663382628119203,-0.244251601209411,
-0.722929908501543));
#11516=CARTESIAN_POINT('Ctrl Pts',(0.631684198665438,-0.232861760990032,
-0.750785745543687));
#11517=CARTESIAN_POINT('Ctrl Pts',(0.615966552324775,-0.224161999508995,
-0.763642258217232));
#11518=CARTESIAN_POINT('Ctrl Pts',(0.587792702767295,-0.203463743702801,
-0.78555112003688));
#11519=CARTESIAN_POINT('Ctrl Pts',(0.573915184558107,-0.190326085855194,
-0.795684265985088));
#11520=CARTESIAN_POINT('Ctrl Pts',(0.548874290046456,-0.159766064500479,
-0.813159949759));
#11521=CARTESIAN_POINT('Ctrl Pts',(0.537715343527944,-0.142345102874864,
-0.820511285096538));
#11522=CARTESIAN_POINT('Ctrl Pts',(0.517157748491652,-0.099930567888331,
-0.833661031856294));
#11523=CARTESIAN_POINT('Ctrl Pts',(0.508899795931835,-0.0740444353928835,
-0.838633903678357));
#11524=CARTESIAN_POINT('Ctrl Pts',(0.504455939115715,-0.04763,-0.841298510752801));
#11525=CARTESIAN_POINT('Origin',(0.707106781186548,-0.04763,-0.707106781186547));
#11526=CARTESIAN_POINT('Origin',(0.,-0.166705,0.));
#11527=CARTESIAN_POINT('',(-0.980948,-0.28578,1.20131482833E-16));
#11528=CARTESIAN_POINT('Origin',(0.,-0.28578,0.));
#11529=CARTESIAN_POINT('',(-0.980948,-0.166705,1.20131482833E-16));
#11530=CARTESIAN_POINT('',(0.951592097314,-0.04763,0.238183666596899));
#11531=CARTESIAN_POINT('Origin',(0.,-0.04763,0.));
#11532=CARTESIAN_POINT('',(0.951592097314,-0.04763,-0.238183666596899));
#11533=CARTESIAN_POINT('Ctrl Pts',(0.951592097314,-0.04763,0.238183666596899));
#11534=CARTESIAN_POINT('Ctrl Pts',(0.952850216871763,-0.0740444353928835,
0.233157223576062));
#11535=CARTESIAN_POINT('Ctrl Pts',(0.955173119738174,-0.099930567888331,
0.223801617934945));
#11536=CARTESIAN_POINT('Ctrl Pts',(0.960411259488514,-0.142345102874864,
0.199966927975188));
#11537=CARTESIAN_POINT('Ctrl Pts',(0.963103647174702,-0.15976606450048,
0.1868781821531));
#11538=CARTESIAN_POINT('Ctrl Pts',(0.968453058988463,-0.190326085855194,
0.15681442133453));
#11539=CARTESIAN_POINT('Ctrl Pts',(0.971100730005489,-0.203463743702801,
0.139836317888042));
#11540=CARTESIAN_POINT('Ctrl Pts',(0.975530745318961,-0.224161999508995,
0.104422493053067));
#11541=CARTESIAN_POINT('Ctrl Pts',(0.977553872336861,-0.232861760990032,
0.0842175114474172));
#11542=CARTESIAN_POINT('Ctrl Pts',(0.980270995488453,-0.244251601209411,
0.0421062857595697));
#11543=CARTESIAN_POINT('Ctrl Pts',(0.980948,-0.246942143572133,0.0201990724523194));
#11544=CARTESIAN_POINT('Ctrl Pts',(0.980948,-0.246942143572133,-0.0201990724523194));
#11545=CARTESIAN_POINT('Ctrl Pts',(0.980270995488453,-0.244251601209411,
-0.0421062857595697));
#11546=CARTESIAN_POINT('Ctrl Pts',(0.977553872336861,-0.232861760990032,
-0.0842175114474172));
#11547=CARTESIAN_POINT('Ctrl Pts',(0.975530745318961,-0.224161999508995,
-0.104422493053067));
#11548=CARTESIAN_POINT('Ctrl Pts',(0.971100730005489,-0.203463743702801,
-0.139836317888042));
#11549=CARTESIAN_POINT('Ctrl Pts',(0.968453058988463,-0.190326085855194,
-0.15681442133453));
#11550=CARTESIAN_POINT('Ctrl Pts',(0.963103647174702,-0.15976606450048,
-0.1868781821531));
#11551=CARTESIAN_POINT('Ctrl Pts',(0.960411259488514,-0.142345102874864,
-0.199966927975188));
#11552=CARTESIAN_POINT('Ctrl Pts',(0.955173119738174,-0.099930567888331,
-0.223801617934945));
#11553=CARTESIAN_POINT('Ctrl Pts',(0.952850216871763,-0.0740444353928835,
-0.233157223576062));
#11554=CARTESIAN_POINT('Ctrl Pts',(0.951592097314,-0.0476299999999999,-0.238183666596899));
#11555=CARTESIAN_POINT('Origin',(0.,-0.04763,0.));
#11556=CARTESIAN_POINT('Origin',(0.,-0.04763,0.));
#11557=CARTESIAN_POINT('Origin',(1.,-0.04763,0.));
#11558=CARTESIAN_POINT('Origin',(1.,0.,0.));
#11559=CARTESIAN_POINT('Origin',(1.,-0.04763,0.));
#11560=CARTESIAN_POINT('Origin',(0.,-0.28578,0.));
#11561=CARTESIAN_POINT('Origin',(0.,-0.04763,0.));
#11694=UNCERTAINTY_MEASURE_WITH_UNIT(LENGTH_MEASURE(0.001),#11749,
'DISTANCE_ACCURACY_VALUE',
'Maximum model space distance between geometric entities at asserted c
onnectivities');
#11699=UNCERTAINTY_MEASURE_WITH_UNIT(LENGTH_MEASURE(0.001),#11749,
'DISTANCE_ACCURACY_VALUE',
'Maximum model space distance between geometric entities at asserted c
onnectivities');
#11743=(
GEOMETRIC_REPRESENTATION_CONTEXT(3)
GLOBAL_UNCERTAINTY_ASSIGNED_CONTEXT((#11694))
GLOBAL_UNIT_ASSIGNED_CONTEXT((#11749,#11751,#11752))
REPRESENTATION_CONTEXT('','3D')
);
#11748=(
GEOMETRIC_REPRESENTATION_CONTEXT(3)
GLOBAL_UNCERTAINTY_ASSIGNED_CONTEXT((#11699))
GLOBAL_UNIT_ASSIGNED_CONTEXT((#11749,#11751,#11752))
REPRESENTATION_CONTEXT('','3D')
);
#11749=(
LENGTH_UNIT()
NAMED_UNIT(*)
SI_UNIT(.CENTI.,.METRE.)
);
#11751=(
NAMED_UNIT(*)
PLANE_ANGLE_UNIT()
SI_UNIT($,.RADIAN.)
);
#11752=(
NAMED_UNIT(*)
SI_UNIT($,.STERADIAN.)
SOLID_ANGLE_UNIT()
);
#11796=SHAPE_DEFINITION_REPRESENTATION(#11904,#11967);
#11904=PRODUCT_DEFINITION_SHAPE('',$,#12016);
#11967=SHAPE_REPRESENTATION('',(#7379),#11743);
#11972=PRODUCT_DEFINITION_CONTEXT('part definition',#12118,'design');
#12016=PRODUCT_DEFINITION('Cage','Cage',#12064,#11972);
#12064=PRODUCT_DEFINITION_FORMATION('',$,#12163);
#12118=APPLICATION_CONTEXT(
'Core Data for Automotive Mechanical Design Process');
#12119=PRODUCT_CONTEXT('part definition',#12118,'mechanical');
#12163=PRODUCT('Cage','Cage','Cage',(#12119));
#12169=PRESENTATION_STYLE_ASSIGNMENT((#12174));
#12174=SURFACE_STYLE_USAGE(.BOTH.,#12179);
#12179=SURFACE_SIDE_STYLE('',(#12184));
#12184=SURFACE_STYLE_FILL_AREA(#12189);
#12189=FILL_AREA_STYLE('CAD Library Painted - Engineering blue',(#12194));
#12194=FILL_AREA_STYLE_COLOUR('CAD Library Painted - Engineering blue',
#12199);
#12199=COLOUR_RGB('CAD Library Painted - Engineering blue',0.12156862745098,
0.356862745098039,0.6);
ENDSEC;
END-ISO-10303-21;
